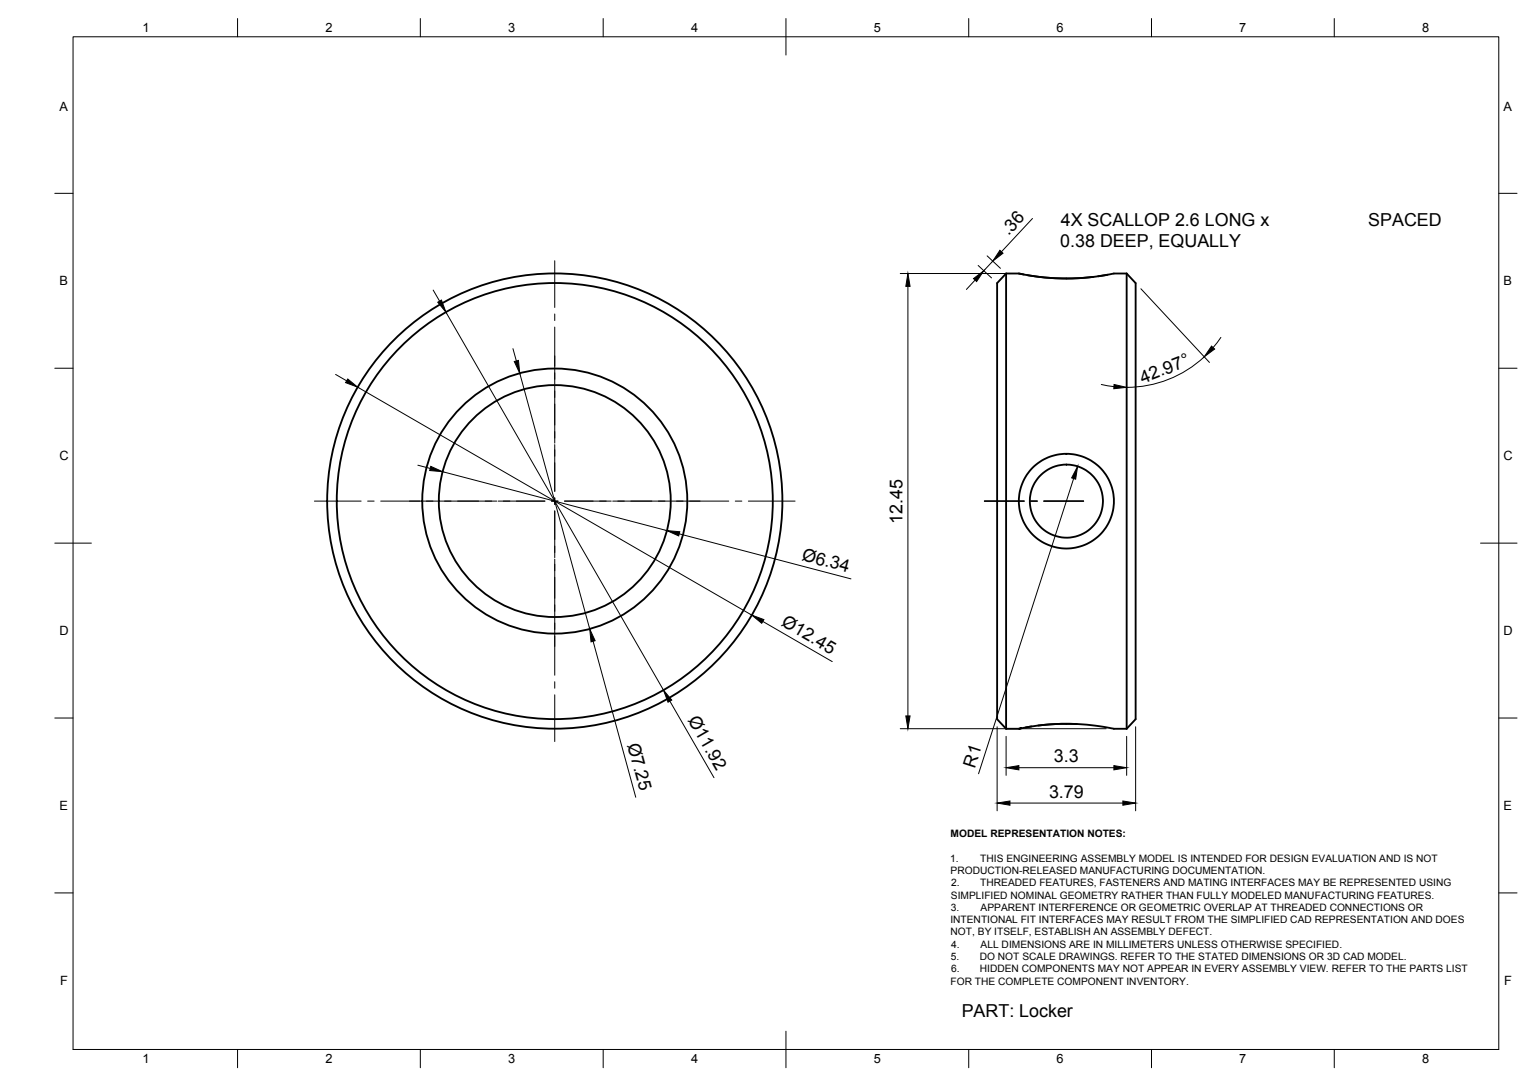
ISO-10303-21;
HEADER;
/* Generated by software containing ST-Developer
 * from STEP Tools, Inc. (www.steptools.com) 
 */

FILE_DESCRIPTION(
/* description */ (''),
/* implementation_level */ '2;1');

FILE_NAME(
/* name */ 'Locker.step',
/* time_stamp */ '2026-10-05T00:51:14-07:00',
/* author */ (''),
/* organization */ (''),
/* preprocessor_version */ 'ST-DEVELOPER v20.2',
/* originating_system */ 'Autodesk Translation Framework v15.15.0.0',
/* authorisation */ '');

FILE_SCHEMA (('AUTOMOTIVE_DESIGN { 1 0 10303 214 3 1 1 }'));
ENDSEC;

DATA;
#10=MECHANICAL_DESIGN_GEOMETRIC_PRESENTATION_REPRESENTATION('',(#392),#4613);
#44=B_SPLINE_SURFACE_WITH_KNOTS('',3,3,((#2717,#2718,#2719,#2720,#2721,
#2722,#2723,#2724,#2725,#2726,#2727,#2728,#2729,#2730,#2731,#2732,#2733,
#2734,#2735,#2736,#2737,#2738,#2739,#2740,#2741,#2742,#2743),(#2744,#2745,
#2746,#2747,#2748,#2749,#2750,#2751,#2752,#2753,#2754,#2755,#2756,#2757,
#2758,#2759,#2760,#2761,#2762,#2763,#2764,#2765,#2766,#2767,#2768,#2769,
#2770),(#2771,#2772,#2773,#2774,#2775,#2776,#2777,#2778,#2779,#2780,#2781,
#2782,#2783,#2784,#2785,#2786,#2787,#2788,#2789,#2790,#2791,#2792,#2793,
#2794,#2795,#2796,#2797),(#2798,#2799,#2800,#2801,#2802,#2803,#2804,#2805,
#2806,#2807,#2808,#2809,#2810,#2811,#2812,#2813,#2814,#2815,#2816,#2817,
#2818,#2819,#2820,#2821,#2822,#2823,#2824)),.UNSPECIFIED.,.F.,.T.,.F.,(4,
4),(4,1,2,1,1,1,2,2,2,2,2,1,1,1,2,2,4),(-9.33776365674593E-5,1.000525980474),
(0.,0.0377394432573701,0.0754788865147403,0.113217461481148,0.150956036447555,
0.188694611413963,0.226433186380371,0.264172629637741,0.301912072895111,
0.339651516152481,0.377390959409851,0.415129534376259,0.452868109342666,
0.490606684309074,0.528345259275481,0.566084702532851,0.603824145790222),
 .UNSPECIFIED.);
#45=B_SPLINE_SURFACE_WITH_KNOTS('',3,3,((#3469,#3470,#3471,#3472,#3473,
#3474,#3475,#3476,#3477,#3478,#3479,#3480,#3481,#3482,#3483,#3484,#3485,
#3486,#3487,#3488,#3489,#3490,#3491,#3492,#3493,#3494,#3495,#3496,#3497),
(#3498,#3499,#3500,#3501,#3502,#3503,#3504,#3505,#3506,#3507,#3508,#3509,
#3510,#3511,#3512,#3513,#3514,#3515,#3516,#3517,#3518,#3519,#3520,#3521,
#3522,#3523,#3524,#3525,#3526),(#3527,#3528,#3529,#3530,#3531,#3532,#3533,
#3534,#3535,#3536,#3537,#3538,#3539,#3540,#3541,#3542,#3543,#3544,#3545,
#3546,#3547,#3548,#3549,#3550,#3551,#3552,#3553,#3554,#3555),(#3556,#3557,
#3558,#3559,#3560,#3561,#3562,#3563,#3564,#3565,#3566,#3567,#3568,#3569,
#3570,#3571,#3572,#3573,#3574,#3575,#3576,#3577,#3578,#3579,#3580,#3581,
#3582,#3583,#3584)),.UNSPECIFIED.,.F.,.T.,.F.,(4,4),(4,1,2,1,2,1,2,2,2,
1,2,1,1,1,1,1,2,2,4),(-0.000295807310057764,1.00205953088178),(0.,0.0377394432573701,
0.0754788865147402,0.113217461481148,0.150956036447555,0.188694611413963,
0.226433186380371,0.264172629637741,0.301912072895111,0.367956098595508,
0.377390959409851,0.415129534376259,0.433998821859462,0.443433465601064,
0.452868109342666,0.490606684309074,0.528345259275481,0.566084702532851,
0.603824145790222),.UNSPECIFIED.);
#46=B_SPLINE_SURFACE_WITH_KNOTS('',3,3,((#3828,#3829,#3830,#3831,#3832,
#3833,#3834,#3835,#3836,#3837,#3838,#3839,#3840,#3841,#3842,#3843,#3844,
#3845,#3846,#3847,#3848,#3849,#3850,#3851,#3852,#3853,#3854),(#3855,#3856,
#3857,#3858,#3859,#3860,#3861,#3862,#3863,#3864,#3865,#3866,#3867,#3868,
#3869,#3870,#3871,#3872,#3873,#3874,#3875,#3876,#3877,#3878,#3879,#3880,
#3881),(#3882,#3883,#3884,#3885,#3886,#3887,#3888,#3889,#3890,#3891,#3892,
#3893,#3894,#3895,#3896,#3897,#3898,#3899,#3900,#3901,#3902,#3903,#3904,
#3905,#3906,#3907,#3908),(#3909,#3910,#3911,#3912,#3913,#3914,#3915,#3916,
#3917,#3918,#3919,#3920,#3921,#3922,#3923,#3924,#3925,#3926,#3927,#3928,
#3929,#3930,#3931,#3932,#3933,#3934,#3935)),.UNSPECIFIED.,.F.,.T.,.F.,(4,
4),(4,1,2,1,1,1,1,2,2,1,1,2,1,1,2,2,2,4),(-0.000127845078603306,1.00073508349094),
(0.,0.0377394432573701,0.0754788865147403,0.113217461481148,0.150956036447555,
0.160390680189157,0.188694611413963,0.226433186380371,0.264172629637741,
0.292477212080768,0.320781794523796,0.377390959409851,0.405694890634657,
0.433998821859462,0.490606684309074,0.528345259275481,0.566084702532852,
0.603824145790222),.UNSPECIFIED.);
#47=B_SPLINE_SURFACE_WITH_KNOTS('',3,3,((#4130,#4131,#4132,#4133,#4134,
#4135,#4136,#4137,#4138,#4139,#4140,#4141,#4142,#4143,#4144,#4145,#4146,
#4147,#4148,#4149,#4150,#4151,#4152,#4153,#4154,#4155,#4156,#4157,#4158,
#4159),(#4160,#4161,#4162,#4163,#4164,#4165,#4166,#4167,#4168,#4169,#4170,
#4171,#4172,#4173,#4174,#4175,#4176,#4177,#4178,#4179,#4180,#4181,#4182,
#4183,#4184,#4185,#4186,#4187,#4188,#4189),(#4190,#4191,#4192,#4193,#4194,
#4195,#4196,#4197,#4198,#4199,#4200,#4201,#4202,#4203,#4204,#4205,#4206,
#4207,#4208,#4209,#4210,#4211,#4212,#4213,#4214,#4215,#4216,#4217,#4218,
#4219),(#4220,#4221,#4222,#4223,#4224,#4225,#4226,#4227,#4228,#4229,#4230,
#4231,#4232,#4233,#4234,#4235,#4236,#4237,#4238,#4239,#4240,#4241,#4242,
#4243,#4244,#4245,#4246,#4247,#4248,#4249)),.UNSPECIFIED.,.F.,.T.,.F.,(4,
4),(4,1,2,1,2,1,2,2,2,2,2,1,1,1,2,2,2,4),(-9.8278797788155E-5,1.00068681548426),
(0.,0.0377394432573701,0.0754788865147402,0.113217461481148,0.150956036447555,
0.188694611413963,0.226433186380371,0.264172629637741,0.301912072895111,
0.339651516152481,0.377390959409851,0.412770873440858,0.433998821859462,
0.462302753084268,0.490606684309074,0.528345259275481,0.566084702532851,
0.603824145790222),.UNSPECIFIED.);
#60=CONICAL_SURFACE('',#1831,6.09377868362497,0.82078898923398);
#61=CONICAL_SURFACE('',#1832,6.09377868362497,0.82078898923398);
#62=CONICAL_SURFACE('',#1836,3.39812786153974,1.04516253667508);
#63=CONICAL_SURFACE('',#1840,3.39812786153974,1.04516253667508);
#84=FACE_BOUND('',#587,.T.);
#85=FACE_BOUND('',#588,.T.);
#86=FACE_BOUND('',#589,.T.);
#87=FACE_BOUND('',#602,.T.);
#88=FACE_BOUND('',#606,.T.);
#114=PLANE('',#1822);
#115=PLANE('',#1823);
#116=PLANE('',#1824);
#117=PLANE('',#1827);
#118=PLANE('',#1828);
#119=PLANE('',#1834);
#139=B_SPLINE_CURVE_WITH_KNOTS('',3,(#2829,#2830,#2831,#2832,#2833,#2834,
#2835,#2836,#2837,#2838,#2839,#2840,#2841,#2842,#2843,#2844,#2845,#2846,
#2847,#2848,#2849,#2850,#2851,#2852,#2853,#2854,#2855,#2856,#2857,#2858,
#2859,#2860,#2861,#2862,#2863,#2864,#2865,#2866,#2867,#2868,#2869,#2870,
#2871,#2872,#2873,#2874,#2875,#2876,#2877,#2878,#2879,#2880,#2881,#2882,
#2883,#2884,#2885,#2886),.UNSPECIFIED.,.F.,.F.,(4,3,3,3,3,3,3,3,3,3,3,3,
3,3,3,3,3,3,3,4),(0.,0.00830256342986541,0.0165421526797814,0.024758238338255,
0.0329694780959283,0.0377394432573701,0.0461457227075515,0.0546067113015583,
0.063111349941413,0.0717202621168138,0.0754788865147403,0.0836526270820083,
0.0917610027075096,0.0998510566328465,0.107954786491979,0.113217461481148,
0.124926744470172,0.136958735315253,0.149276745375588,0.150956036447555),
 .UNSPECIFIED.);
#140=B_SPLINE_CURVE_WITH_KNOTS('',3,(#2887,#2888,#2889,#2890,#2891,#2892,
#2893,#2894,#2895,#2896,#2897,#2898,#2899,#2900,#2901,#2902,#2903,#2904,
#2905,#2906,#2907,#2908),.UNSPECIFIED.,.F.,.F.,(4,1,2,2,2,2,2,1,1,1,2,2,
4),(0.150956036447555,0.188694611413963,0.226433186380371,0.264172629637741,
0.301912072895111,0.339651516152481,0.377390959409851,0.415129534376259,
0.452868109342666,0.490606684309074,0.528345259275481,0.566084702532851,
0.603824145790222),.UNSPECIFIED.);
#141=B_SPLINE_CURVE_WITH_KNOTS('',3,(#2910,#2911,#2912,#2913,#2914,#2915,
#2916,#2917,#2918,#2919,#2920,#2921,#2922,#2923,#2924,#2925,#2926,#2927),
 .UNSPECIFIED.,.F.,.F.,(4,2,2,2,2,2,2,2,4),(0.,0.0225535375719625,0.045742561528813,
0.0614467959049737,0.0822737875323286,0.105553304717535,0.131394096503778,
0.166373424514803,0.179386291539105),.UNSPECIFIED.);
#142=B_SPLINE_CURVE_WITH_KNOTS('',3,(#2929,#2930,#2931,#2932,#2933,#2934,
#2935,#2936,#2937,#2938,#2939,#2940,#2941,#2942,#2943,#2944,#2945,#2946,
#2947,#2948,#2949,#2950,#2951,#2952,#2953,#2954,#2955,#2956,#2957,#2958,
#2959,#2960),.UNSPECIFIED.,.F.,.F.,(4,2,2,2,2,2,2,2,2,2,2,2,2,2,2,4),(0.179386291539105,
0.180187796446041,0.193753938234979,0.227654303126555,0.255593035139534,
0.354710269922964,0.40331380346349,0.454831190769845,0.497871745499511,
0.537911247906565,0.557044545701239,0.596336621939663,0.650672125427441,
0.738536442549073,0.86973485948851,1.00167935296521),.UNSPECIFIED.);
#143=B_SPLINE_CURVE_WITH_KNOTS('',3,(#2961,#2962,#2963,#2964,#2965,#2966,
#2967,#2968,#2969,#2970,#2971,#2972,#2973,#2974),.UNSPECIFIED.,.F.,.F.,
(4,2,2,2,2,2,4),(2.12484122892953E-5,0.0384114166919255,0.0840005064200764,
0.134083217100535,0.322530315130806,0.421641395496061,0.518312663440211),
 .UNSPECIFIED.);
#144=B_SPLINE_CURVE_WITH_KNOTS('',3,(#2983,#2984,#2985,#2986,#2987,#2988,
#2989,#2990,#2991,#2992,#2993,#2994,#2995,#2996,#2997,#2998,#2999,#3000,
#3001,#3002,#3003,#3004,#3005,#3006,#3007,#3008,#3009,#3010,#3011,#3012,
#3013,#3014,#3015,#3016,#3017,#3018,#3019,#3020,#3021,#3022,#3023,#3024,
#3025,#3026,#3027,#3028,#3029,#3030,#3031,#3032,#3033,#3034,#3035,#3036,
#3037,#3038,#3039,#3040,#3041,#3042,#3043,#3044,#3045,#3046,#3047,#3048,
#3049,#3050,#3051,#3052,#3053,#3054,#3055,#3056,#3057,#3058,#3059,#3060,
#3061,#3062,#3063,#3064,#3065,#3066,#3067,#3068,#3069,#3070,#3071,#3072,
#3073,#3074,#3075,#3076,#3077,#3078,#3079,#3080,#3081,#3082,#3083,#3084,
#3085,#3086,#3087,#3088,#3089,#3090,#3091,#3092,#3093,#3094,#3095,#3096,
#3097,#3098,#3099,#3100,#3101,#3102,#3103,#3104,#3105,#3106,#3107,#3108,
#3109,#3110,#3111,#3112,#3113,#3114,#3115,#3116,#3117,#3118,#3119,#3120,
#3121,#3122,#3123,#3124,#3125,#3126,#3127,#3128,#3129,#3130,#3131,#3132,
#3133,#3134,#3135,#3136,#3137,#3138,#3139,#3140,#3141,#3142,#3143,#3144,
#3145,#3146,#3147,#3148),.UNSPECIFIED.,.T.,.F.,(4,3,3,3,3,3,3,3,3,3,3,3,
3,3,3,3,3,3,3,3,3,3,3,3,3,3,3,3,3,3,3,3,3,3,3,3,3,3,3,3,3,3,3,3,3,3,3,3,
3,3,3,3,3,3,3,4),(-0.603824145790222,-0.590391584697042,-0.577063699872746,
-0.566084702532851,-0.547214980904166,-0.533196018247437,-0.528345259275481,
-0.514141540772843,-0.5016291634541,-0.490606684309074,-0.479313082523423,
-0.468129273627917,-0.456937255878014,-0.452868109342666,-0.44488880016883,
-0.443433465601064,-0.43506567000572,-0.433998821859462,-0.422340513015576,
-0.415129534376259,-0.402742107601763,-0.388956278039157,-0.377390959409851,
-0.368495774245557,-0.367956098595508,-0.35039657661204,-0.334829325286879,
-0.320458700988321,-0.307238340240676,-0.301912072895111,-0.288351696410483,
-0.275229547002117,-0.264172629637741,-0.245302908009056,-0.231165617978299,
-0.226433186380371,-0.211738883366401,-0.19886806654317,-0.188694611413963,
-0.177840892685696,-0.167083403070668,-0.156287372800931,-0.150956036447555,
-0.140167573510221,-0.129416044354867,-0.118538583805277,-0.113217461481148,
-0.100521490014891,-0.0863362768838805,-0.0754788865147402,-0.0614072540763898,
-0.0441325663214528,-0.0377394432573701,-0.0243206710161803,-0.0108972336665805,
0.),.UNSPECIFIED.);
#145=B_SPLINE_CURVE_WITH_KNOTS('',3,(#3150,#3151,#3152,#3153,#3154,#3155,
#3156,#3157,#3158,#3159,#3160,#3161,#3162,#3163,#3164,#3165,#3166,#3167,
#3168,#3169,#3170,#3171,#3172,#3173,#3174,#3175,#3176,#3177,#3178,#3179,
#3180,#3181,#3182,#3183,#3184,#3185,#3186,#3187,#3188,#3189,#3190,#3191,
#3192,#3193,#3194,#3195,#3196,#3197,#3198,#3199,#3200,#3201,#3202,#3203,
#3204,#3205,#3206,#3207,#3208,#3209,#3210,#3211,#3212,#3213,#3214,#3215,
#3216,#3217,#3218,#3219,#3220,#3221,#3222,#3223,#3224,#3225,#3226,#3227,
#3228,#3229,#3230,#3231,#3232,#3233,#3234,#3235,#3236,#3237,#3238,#3239,
#3240,#3241,#3242,#3243,#3244,#3245,#3246,#3247,#3248,#3249,#3250,#3251,
#3252,#3253,#3254,#3255,#3256,#3257,#3258,#3259,#3260,#3261,#3262,#3263,
#3264,#3265,#3266,#3267,#3268,#3269,#3270,#3271,#3272,#3273,#3274,#3275,
#3276,#3277,#3278,#3279,#3280,#3281,#3282,#3283,#3284,#3285,#3286,#3287,
#3288,#3289,#3290,#3291,#3292,#3293,#3294,#3295,#3296,#3297,#3298,#3299,
#3300,#3301,#3302,#3303,#3304,#3305,#3306),.UNSPECIFIED.,.T.,.F.,(4,3,3,
3,3,3,3,3,3,3,3,3,3,3,3,3,3,3,3,3,3,3,3,3,3,3,3,3,3,3,3,3,3,3,3,3,3,3,3,
3,3,3,3,3,3,3,3,3,3,3,3,3,4),(-0.603824145790222,-0.59040484149205,-0.577046286087289,
-0.566084702532851,-0.547214980904166,-0.533215939038458,-0.528345259275481,
-0.513405700683712,-0.500371614295665,-0.490606684309074,-0.479523112948318,
-0.468575947550825,-0.462302753084268,-0.448150787471865,-0.433998821859462,
-0.424198693428956,-0.414259352480831,-0.412770873440858,-0.398547629668401,
-0.382168241492649,-0.377390959409851,-0.363265067662413,-0.345806810116418,
-0.339651516152481,-0.326317147459025,-0.312908174453228,-0.301912072895111,
-0.288487301763661,-0.2751501468201,-0.264172629637741,-0.245302908009056,
-0.231228232357298,-0.226433186380371,-0.2117347177624,-0.198863361209748,
-0.188694611413963,-0.177846084312265,-0.167093676385978,-0.15630237051341,
-0.150956036447555,-0.140168989421454,-0.129419180679109,-0.118543795278154,
-0.113217461481148,-0.10052665633752,-0.0863472586539609,-0.0754788865147402,
-0.0614129693111486,-0.0441577717811917,-0.0377394432573701,-0.0243211983180093,
-0.0108969351998749,0.),.UNSPECIFIED.);
#146=B_SPLINE_CURVE_WITH_KNOTS('',3,(#3308,#3309,#3310,#3311,#3312,#3313,
#3314,#3315,#3316,#3317,#3318,#3319,#3320,#3321,#3322,#3323,#3324,#3325,
#3326,#3327,#3328,#3329,#3330,#3331,#3332,#3333,#3334,#3335,#3336,#3337,
#3338,#3339,#3340,#3341,#3342,#3343,#3344,#3345,#3346,#3347,#3348,#3349,
#3350,#3351,#3352,#3353,#3354,#3355,#3356,#3357,#3358,#3359,#3360,#3361,
#3362,#3363,#3364,#3365,#3366,#3367,#3368,#3369,#3370,#3371,#3372,#3373,
#3374,#3375,#3376,#3377,#3378,#3379,#3380,#3381,#3382,#3383,#3384,#3385,
#3386,#3387,#3388,#3389,#3390,#3391,#3392,#3393,#3394,#3395,#3396,#3397,
#3398,#3399,#3400,#3401,#3402,#3403,#3404,#3405,#3406,#3407,#3408,#3409,
#3410,#3411,#3412,#3413,#3414,#3415,#3416,#3417,#3418,#3419,#3420,#3421,
#3422,#3423,#3424,#3425,#3426,#3427,#3428,#3429,#3430,#3431,#3432,#3433,
#3434,#3435,#3436,#3437,#3438,#3439,#3440,#3441,#3442,#3443,#3444,#3445,
#3446,#3447,#3448,#3449,#3450,#3451,#3452,#3453,#3454,#3455,#3456,#3457,
#3458,#3459,#3460,#3461,#3462,#3463,#3464),.UNSPECIFIED.,.T.,.F.,(4,3,3,
3,3,3,3,3,3,3,3,3,3,3,3,3,3,3,3,3,3,3,3,3,3,3,3,3,3,3,3,3,3,3,3,3,3,3,3,
3,3,3,3,3,3,3,3,3,3,3,3,3,4),(-0.603824145790222,-0.590411465612469,-0.577041801624018,
-0.566084702532852,-0.547214980904167,-0.533151553554515,-0.528345259275481,
-0.511854870778258,-0.497832584846173,-0.490606684309074,-0.473210539692822,
-0.455925683856001,-0.438701796249427,-0.433998821859462,-0.423201659387045,
-0.412132127313061,-0.405694890634657,-0.390813405226797,-0.377390959409851,
-0.359294156561789,-0.340037975542793,-0.32497088632671,-0.320781794523796,
-0.307843399048729,-0.294273409598876,-0.292477212080768,-0.279144117317815,
-0.266288363724764,-0.264172629637741,-0.245302908009056,-0.231166470585065,
-0.226433186380371,-0.210823746419028,-0.197307415534654,-0.188694611413963,
-0.178396491003475,-0.168205689857489,-0.160390680189157,-0.15167832823336,
-0.150956036447555,-0.139587056809165,-0.128218450390218,-0.116689538696443,
-0.113217461481148,-0.100992605061081,-0.0874389990760216,-0.0754788865147403,
-0.0614233370420267,-0.0442069385936118,-0.0377394432573701,-0.0243181691647032,
-0.010894129954878,0.),.UNSPECIFIED.);
#147=B_SPLINE_CURVE_WITH_KNOTS('',3,(#3588,#3589,#3590,#3591,#3592,#3593,
#3594,#3595,#3596,#3597,#3598,#3599,#3600,#3601,#3602,#3603,#3604,#3605,
#3606,#3607,#3608,#3609,#3610,#3611,#3612,#3613,#3614,#3615,#3616,#3617,
#3618,#3619,#3620,#3621,#3622,#3623,#3624,#3625,#3626,#3627,#3628,#3629,
#3630,#3631,#3632,#3633,#3634,#3635,#3636,#3637,#3638,#3639,#3640,#3641,
#3642,#3643,#3644,#3645),.UNSPECIFIED.,.F.,.F.,(4,3,3,3,3,3,3,3,3,3,3,3,
3,3,3,3,3,3,3,4),(0.,0.00829573762667763,0.0165281897599753,0.0247370376512881,
0.0329409858379027,0.0377394432573701,0.0462233213317535,0.0547599525540828,
0.0633384602639499,0.0720158188648333,0.0754788865147402,0.0849135302563422,
0.0940108607641121,0.103092592101262,0.112175512163797,0.113217461481148,
0.122710740047244,0.132228579300877,0.141826740872809,0.150956036447555),
 .UNSPECIFIED.);
#148=B_SPLINE_CURVE_WITH_KNOTS('',3,(#3646,#3647,#3648,#3649,#3650,#3651,
#3652,#3653,#3654,#3655,#3656,#3657,#3658,#3659,#3660,#3661,#3662,#3663,
#3664,#3665,#3666,#3667,#3668,#3669,#3670,#3671,#3672,#3673,#3674,#3675,
#3676,#3677,#3678,#3679,#3680,#3681,#3682,#3683,#3684,#3685,#3686,#3687,
#3688,#3689,#3690,#3691,#3692,#3693,#3694,#3695,#3696,#3697,#3698,#3699,
#3700,#3701,#3702,#3703,#3704,#3705,#3706,#3707,#3708,#3709,#3710,#3711,
#3712,#3713,#3714,#3715,#3716,#3717,#3718,#3719,#3720,#3721,#3722,#3723,
#3724,#3725,#3726,#3727,#3728,#3729,#3730,#3731,#3732,#3733,#3734,#3735,
#3736,#3737,#3738,#3739,#3740,#3741,#3742,#3743,#3744,#3745,#3746,#3747,
#3748,#3749,#3750,#3751,#3752,#3753,#3754,#3755,#3756,#3757,#3758,#3759,
#3760,#3761,#3762,#3763,#3764,#3765,#3766,#3767,#3768,#3769,#3770,#3771,
#3772,#3773,#3774,#3775,#3776,#3777,#3778,#3779,#3780,#3781,#3782,#3783,
#3784,#3785,#3786,#3787,#3788,#3789,#3790,#3791,#3792,#3793,#3794,#3795,
#3796,#3797,#3798,#3799,#3800,#3801,#3802,#3803,#3804,#3805,#3806,#3807,
#3808,#3809,#3810,#3811,#3812,#3813,#3814,#3815,#3816,#3817,#3818,#3819,
#3820,#3821,#3822,#3823),.UNSPECIFIED.,.F.,.F.,(4,3,3,3,3,3,3,3,3,3,3,3,
3,3,3,3,3,3,3,3,3,3,3,3,3,3,3,3,3,3,3,3,3,3,3,3,3,3,3,3,3,3,3,3,3,3,3,3,
3,3,3,3,3,3,3,3,3,3,3,4),(0.150956036447555,0.160549363754181,0.170087496495515,
0.17957549259755,0.188694611413963,0.198129255155565,0.20721232152291,0.216307090036003,
0.225442296384496,0.226433186380371,0.235263130335913,0.243982144413462,
0.252652316208085,0.261280881376461,0.264172629637741,0.272628973289914,
0.281096319050457,0.289577868539869,0.298109252272672,0.301912072895111,
0.310541878044286,0.3191353238789,0.327707744142598,0.336272944326547,0.344860159102294,
0.35346693169753,0.362137437500319,0.367956098595508,0.375378363711079,
0.377390959409851,0.386825603151453,0.395781405680958,0.404721766264308,
0.413665159126656,0.415129534376259,0.426960243388473,0.433998821859462,
0.440518945174589,0.443433465601064,0.449108910733518,0.452868109342666,
0.463354416125425,0.473794794225623,0.484190742563337,0.490606684309074,
0.499415552802534,0.508224959525105,0.517045112657598,0.525909821728332,
0.528345259275481,0.537116996273335,0.545776074243873,0.554386030522553,
0.562954515301158,0.566084702532851,0.574305585613258,0.582536335557294,
0.590782316872269,0.59908512911533,0.603824145790222),.UNSPECIFIED.);
#149=B_SPLINE_CURVE_WITH_KNOTS('',3,(#3939,#3940,#3941,#3942,#3943,#3944,
#3945,#3946,#3947,#3948,#3949,#3950,#3951,#3952,#3953,#3954,#3955,#3956),
 .UNSPECIFIED.,.F.,.F.,(4,2,2,2,2,2,2,2,4),(-0.157966795349973,-0.134769746245384,
-0.111152103192473,-0.0957393456100155,-0.0764377111352473,-0.0499851580328299,
-0.0372293294602945,-0.0183607331665397,-1.54852585271355E-5),
 .UNSPECIFIED.);
#150=B_SPLINE_CURVE_WITH_KNOTS('',3,(#3957,#3958,#3959,#3960,#3961,#3962,
#3963,#3964,#3965,#3966,#3967,#3968,#3969,#3970,#3971,#3972,#3973,#3974,
#3975,#3976,#3977,#3978,#3979,#3980,#3981,#3982,#3983,#3984,#3985,#3986,
#3987,#3988,#3989,#3990,#3991,#3992,#3993,#3994,#3995,#3996,#3997,#3998,
#3999,#4000,#4001,#4002,#4003,#4004,#4005,#4006,#4007,#4008,#4009,#4010,
#4011,#4012,#4013,#4014,#4015,#4016,#4017,#4018,#4019,#4020,#4021,#4022,
#4023,#4024,#4025,#4026,#4027,#4028,#4029,#4030,#4031,#4032,#4033,#4034,
#4035,#4036,#4037,#4038,#4039,#4040,#4041,#4042,#4043,#4044,#4045,#4046,
#4047,#4048,#4049,#4050,#4051,#4052,#4053,#4054,#4055,#4056,#4057,#4058,
#4059,#4060,#4061,#4062,#4063,#4064,#4065,#4066,#4067,#4068,#4069,#4070,
#4071,#4072,#4073,#4074,#4075,#4076,#4077,#4078,#4079,#4080,#4081,#4082,
#4083,#4084,#4085,#4086,#4087,#4088,#4089,#4090,#4091,#4092,#4093,#4094,
#4095,#4096,#4097,#4098,#4099,#4100,#4101,#4102,#4103,#4104,#4105,#4106,
#4107,#4108,#4109,#4110,#4111,#4112,#4113,#4114,#4115,#4116,#4117,#4118,
#4119,#4120,#4121,#4122),.UNSPECIFIED.,.F.,.F.,(4,3,3,3,3,3,3,3,3,3,3,3,
3,3,3,3,3,3,3,3,3,3,3,3,3,3,3,3,3,3,3,3,3,3,3,3,3,3,3,3,3,3,3,3,3,3,3,3,
3,3,3,3,3,3,3,4),(0.150956046102631,0.157057308185334,0.160390680189157,
0.169102327349017,0.177761740636142,0.186381822627463,0.188694611413963,
0.198129255155565,0.207504363975699,0.216968775178035,0.226433186380371,
0.235339806064433,0.244136369675249,0.252883841436447,0.26158882295505,
0.264172629637741,0.273921145643219,0.283689652217834,0.292477212080768,
0.301909496950062,0.311349416446087,0.320781794523796,0.328948709583596,
0.33710056797636,0.345254117291374,0.353452734644994,0.361688284787263,
0.37003334621096,0.377390959409851,0.385901375718853,0.394375368564309,
0.402830843321504,0.405694890634657,0.415170724108714,0.424683263298954,
0.433998821859462,0.443965968418747,0.454061131183995,0.46415325099199,
0.474130092027922,0.483814161418412,0.490606684309074,0.500095510584781,
0.509588520092461,0.519121097655791,0.528345259275481,0.537152260065718,
0.545849424317997,0.554498405743932,0.563106711158609,0.566084702532852,
0.574301473245816,0.582528508095237,0.590771006435055,0.599070784708944,
0.603824145790222),.UNSPECIFIED.);
#151=B_SPLINE_CURVE_WITH_KNOTS('',3,(#4253,#4254,#4255,#4256,#4257,#4258,
#4259,#4260,#4261,#4262,#4263,#4264,#4265,#4266,#4267,#4268,#4269,#4270,
#4271,#4272),.UNSPECIFIED.,.F.,.F.,(4,2,2,2,2,2,2,2,2,4),(-0.63257270273012,
-0.613187885769762,-0.594110099534741,-0.574392662092664,-0.55480528669817,
-0.535546049297075,-0.516021545010237,-0.496492553321205,-0.477063998339651,
-0.474227533561733),.UNSPECIFIED.);
#152=B_SPLINE_CURVE_WITH_KNOTS('',3,(#4273,#4274,#4275,#4276,#4277,#4278,
#4279,#4280,#4281,#4282,#4283,#4284,#4285,#4286,#4287,#4288,#4289,#4290,
#4291,#4292,#4293,#4294,#4295,#4296,#4297,#4298,#4299,#4300,#4301,#4302,
#4303,#4304,#4305,#4306,#4307,#4308,#4309,#4310,#4311,#4312,#4313,#4314,
#4315,#4316,#4317,#4318,#4319,#4320,#4321,#4322,#4323,#4324),
 .UNSPECIFIED.,.F.,.F.,(4,2,2,2,2,2,2,2,2,2,2,2,2,2,2,2,2,2,2,2,2,2,2,2,
2,4),(-0.474227533561733,-0.458329372527362,-0.439173439486182,-0.419731155843369,
-0.400140639763559,-0.381254494509653,-0.362129574615996,-0.342849277390761,
-0.315940533098414,-0.289017768986139,-0.269733478910581,-0.250586364422205,
-0.231653812692583,-0.21172855838034,-0.201929598171686,-0.182564500685825,
-0.163995370742465,-0.144570150007686,-0.125002244985411,-0.105396599383871,
-0.0956567919090896,-0.0764809925540918,-0.0569765610843296,-0.0373737466489288,
-0.0184652873791742,0.),.UNSPECIFIED.);
#205=LINE('',#2827,#288);
#206=LINE('',#2978,#289);
#207=LINE('',#2980,#290);
#208=LINE('',#3468,#291);
#209=LINE('',#3586,#292);
#210=LINE('',#3827,#293);
#211=LINE('',#3937,#294);
#212=LINE('',#4126,#295);
#213=LINE('',#4251,#296);
#214=LINE('',#4328,#297);
#215=LINE('',#4336,#298);
#216=LINE('',#4339,#299);
#217=LINE('',#4347,#300);
#218=LINE('',#4351,#301);
#219=LINE('',#4353,#302);
#288=VECTOR('',#2186,10.);
#289=VECTOR('',#2191,6.22506754791384);
#290=VECTOR('',#2192,6.22506754791384);
#291=VECTOR('',#2199,1.);
#292=VECTOR('',#2200,9.99999999999999);
#293=VECTOR('',#2205,1.);
#294=VECTOR('',#2206,10.);
#295=VECTOR('',#2211,1.);
#296=VECTOR('',#2218,10.);
#297=VECTOR('',#2223,1.);
#298=VECTOR('',#2234,6.09377868362497);
#299=VECTOR('',#2237,6.09377868362497);
#300=VECTOR('',#2248,3.39812786153974);
#301=VECTOR('',#2253,3.17127539348974);
#302=VECTOR('',#2256,3.39812786153974);
#354=CYLINDRICAL_SURFACE('',#1813,6.22506754791384);
#355=CYLINDRICAL_SURFACE('',#1816,1.);
#356=CYLINDRICAL_SURFACE('',#1818,1.);
#357=CYLINDRICAL_SURFACE('',#1820,1.);
#358=CYLINDRICAL_SURFACE('',#1825,1.);
#359=CYLINDRICAL_SURFACE('',#1838,3.17127539348974);
#376=SHAPE_REPRESENTATION_RELATIONSHIP('SRR','None',#4650,#384);
#384=ADVANCED_BREP_SHAPE_REPRESENTATION('',(#400),#4610);
#392=STYLED_ITEM('',(#4695),#400);
#400=MANIFOLD_SOLID_BREP('Body1',#1599);
#462=FACE_OUTER_BOUND('',#585,.T.);
#463=FACE_OUTER_BOUND('',#586,.T.);
#464=FACE_OUTER_BOUND('',#590,.T.);
#465=FACE_OUTER_BOUND('',#591,.T.);
#466=FACE_OUTER_BOUND('',#592,.T.);
#467=FACE_OUTER_BOUND('',#593,.T.);
#468=FACE_OUTER_BOUND('',#594,.T.);
#469=FACE_OUTER_BOUND('',#595,.T.);
#470=FACE_OUTER_BOUND('',#596,.T.);
#471=FACE_OUTER_BOUND('',#597,.T.);
#472=FACE_OUTER_BOUND('',#598,.T.);
#473=FACE_OUTER_BOUND('',#599,.T.);
#474=FACE_OUTER_BOUND('',#600,.T.);
#475=FACE_OUTER_BOUND('',#601,.T.);
#476=FACE_OUTER_BOUND('',#603,.T.);
#477=FACE_OUTER_BOUND('',#604,.T.);
#478=FACE_OUTER_BOUND('',#605,.T.);
#479=FACE_OUTER_BOUND('',#607,.T.);
#480=FACE_OUTER_BOUND('',#608,.T.);
#481=FACE_OUTER_BOUND('',#609,.T.);
#585=EDGE_LOOP('',(#1277,#1278,#1279,#1280,#1281,#1282,#1283));
#586=EDGE_LOOP('',(#1284,#1285,#1286,#1287,#1288,#1289,#1290,#1291,#1292));
#587=EDGE_LOOP('',(#1293));
#588=EDGE_LOOP('',(#1294));
#589=EDGE_LOOP('',(#1295));
#590=EDGE_LOOP('',(#1296,#1297,#1298,#1299,#1300));
#591=EDGE_LOOP('',(#1301,#1302,#1303,#1304,#1305));
#592=EDGE_LOOP('',(#1306,#1307,#1308,#1309,#1310));
#593=EDGE_LOOP('',(#1311,#1312,#1313,#1314,#1315));
#594=EDGE_LOOP('',(#1316,#1317,#1318,#1319,#1320));
#595=EDGE_LOOP('',(#1321));
#596=EDGE_LOOP('',(#1322));
#597=EDGE_LOOP('',(#1323));
#598=EDGE_LOOP('',(#1324,#1325,#1326,#1327,#1328));
#599=EDGE_LOOP('',(#1329,#1330,#1331,#1332,#1333));
#600=EDGE_LOOP('',(#1334));
#601=EDGE_LOOP('',(#1335));
#602=EDGE_LOOP('',(#1336));
#603=EDGE_LOOP('',(#1337,#1338,#1339,#1340));
#604=EDGE_LOOP('',(#1341,#1342,#1343,#1344));
#605=EDGE_LOOP('',(#1345));
#606=EDGE_LOOP('',(#1346));
#607=EDGE_LOOP('',(#1347,#1348,#1349,#1350));
#608=EDGE_LOOP('',(#1351,#1352,#1353,#1354));
#609=EDGE_LOOP('',(#1355,#1356,#1357,#1358));
#695=CIRCLE('',#1814,6.22506754791384);
#696=CIRCLE('',#1815,6.22506754791384);
#697=CIRCLE('',#1817,1.);
#698=CIRCLE('',#1819,1.);
#699=CIRCLE('',#1821,1.);
#700=CIRCLE('',#1826,1.);
#701=CIRCLE('',#1829,5.96248981933611);
#702=CIRCLE('',#1830,3.62498032958974);
#703=CIRCLE('',#1833,5.96248981933611);
#704=CIRCLE('',#1835,3.62498032958974);
#705=CIRCLE('',#1837,3.17127539348974);
#706=CIRCLE('',#1839,3.17127539348974);
#796=VERTEX_POINT('',#2825);
#797=VERTEX_POINT('',#2826);
#798=VERTEX_POINT('',#2828);
#799=VERTEX_POINT('',#2909);
#800=VERTEX_POINT('',#2928);
#801=VERTEX_POINT('',#2976);
#802=VERTEX_POINT('',#2979);
#803=VERTEX_POINT('',#2982);
#804=VERTEX_POINT('',#3149);
#805=VERTEX_POINT('',#3307);
#806=VERTEX_POINT('',#3466);
#807=VERTEX_POINT('',#3585);
#808=VERTEX_POINT('',#3587);
#809=VERTEX_POINT('',#3825);
#810=VERTEX_POINT('',#3936);
#811=VERTEX_POINT('',#3938);
#812=VERTEX_POINT('',#4124);
#813=VERTEX_POINT('',#4250);
#814=VERTEX_POINT('',#4252);
#815=VERTEX_POINT('',#4326);
#816=VERTEX_POINT('',#4331);
#817=VERTEX_POINT('',#4333);
#818=VERTEX_POINT('',#4338);
#819=VERTEX_POINT('',#4342);
#820=VERTEX_POINT('',#4345);
#821=VERTEX_POINT('',#4349);
#966=EDGE_CURVE('',#796,#797,#205,.T.);
#967=EDGE_CURVE('',#797,#798,#139,.T.);
#968=EDGE_CURVE('',#798,#797,#140,.T.);
#969=EDGE_CURVE('',#796,#799,#141,.T.);
#970=EDGE_CURVE('',#799,#800,#142,.T.);
#971=EDGE_CURVE('',#800,#796,#143,.T.);
#972=EDGE_CURVE('',#801,#801,#695,.T.);
#973=EDGE_CURVE('',#801,#799,#206,.T.);
#974=EDGE_CURVE('',#800,#802,#207,.T.);
#975=EDGE_CURVE('',#802,#802,#696,.T.);
#976=EDGE_CURVE('',#803,#803,#144,.T.);
#977=EDGE_CURVE('',#804,#804,#145,.T.);
#978=EDGE_CURVE('',#805,#805,#146,.T.);
#979=EDGE_CURVE('',#806,#806,#697,.T.);
#980=EDGE_CURVE('',#806,#798,#208,.T.);
#981=EDGE_CURVE('',#803,#807,#209,.T.);
#982=EDGE_CURVE('',#807,#808,#147,.T.);
#983=EDGE_CURVE('',#808,#807,#148,.T.);
#984=EDGE_CURVE('',#809,#809,#698,.T.);
#985=EDGE_CURVE('',#809,#808,#210,.T.);
#986=EDGE_CURVE('',#805,#810,#211,.T.);
#987=EDGE_CURVE('',#810,#811,#149,.T.);
#988=EDGE_CURVE('',#811,#810,#150,.T.);
#989=EDGE_CURVE('',#812,#812,#699,.T.);
#990=EDGE_CURVE('',#812,#811,#212,.T.);
#991=EDGE_CURVE('',#804,#813,#213,.T.);
#992=EDGE_CURVE('',#813,#814,#151,.T.);
#993=EDGE_CURVE('',#814,#813,#152,.T.);
#994=EDGE_CURVE('',#815,#815,#700,.T.);
#995=EDGE_CURVE('',#815,#814,#214,.T.);
#996=EDGE_CURVE('',#816,#816,#701,.T.);
#997=EDGE_CURVE('',#817,#817,#702,.T.);
#998=EDGE_CURVE('',#802,#816,#215,.T.);
#999=EDGE_CURVE('',#801,#818,#216,.T.);
#1000=EDGE_CURVE('',#818,#818,#703,.T.);
#1001=EDGE_CURVE('',#819,#819,#704,.T.);
#1002=EDGE_CURVE('',#820,#820,#705,.T.);
#1003=EDGE_CURVE('',#820,#819,#217,.T.);
#1004=EDGE_CURVE('',#821,#821,#706,.T.);
#1005=EDGE_CURVE('',#821,#820,#218,.T.);
#1006=EDGE_CURVE('',#821,#817,#219,.T.);
#1277=ORIENTED_EDGE('',*,*,#966,.T.);
#1278=ORIENTED_EDGE('',*,*,#967,.T.);
#1279=ORIENTED_EDGE('',*,*,#968,.T.);
#1280=ORIENTED_EDGE('',*,*,#966,.F.);
#1281=ORIENTED_EDGE('',*,*,#969,.T.);
#1282=ORIENTED_EDGE('',*,*,#970,.T.);
#1283=ORIENTED_EDGE('',*,*,#971,.T.);
#1284=ORIENTED_EDGE('',*,*,#972,.F.);
#1285=ORIENTED_EDGE('',*,*,#973,.T.);
#1286=ORIENTED_EDGE('',*,*,#969,.F.);
#1287=ORIENTED_EDGE('',*,*,#971,.F.);
#1288=ORIENTED_EDGE('',*,*,#974,.T.);
#1289=ORIENTED_EDGE('',*,*,#975,.T.);
#1290=ORIENTED_EDGE('',*,*,#974,.F.);
#1291=ORIENTED_EDGE('',*,*,#970,.F.);
#1292=ORIENTED_EDGE('',*,*,#973,.F.);
#1293=ORIENTED_EDGE('',*,*,#976,.F.);
#1294=ORIENTED_EDGE('',*,*,#977,.F.);
#1295=ORIENTED_EDGE('',*,*,#978,.F.);
#1296=ORIENTED_EDGE('',*,*,#979,.F.);
#1297=ORIENTED_EDGE('',*,*,#980,.T.);
#1298=ORIENTED_EDGE('',*,*,#967,.F.);
#1299=ORIENTED_EDGE('',*,*,#968,.F.);
#1300=ORIENTED_EDGE('',*,*,#980,.F.);
#1301=ORIENTED_EDGE('',*,*,#981,.T.);
#1302=ORIENTED_EDGE('',*,*,#982,.T.);
#1303=ORIENTED_EDGE('',*,*,#983,.T.);
#1304=ORIENTED_EDGE('',*,*,#981,.F.);
#1305=ORIENTED_EDGE('',*,*,#976,.T.);
#1306=ORIENTED_EDGE('',*,*,#984,.F.);
#1307=ORIENTED_EDGE('',*,*,#985,.T.);
#1308=ORIENTED_EDGE('',*,*,#982,.F.);
#1309=ORIENTED_EDGE('',*,*,#983,.F.);
#1310=ORIENTED_EDGE('',*,*,#985,.F.);
#1311=ORIENTED_EDGE('',*,*,#986,.T.);
#1312=ORIENTED_EDGE('',*,*,#987,.T.);
#1313=ORIENTED_EDGE('',*,*,#988,.T.);
#1314=ORIENTED_EDGE('',*,*,#986,.F.);
#1315=ORIENTED_EDGE('',*,*,#978,.T.);
#1316=ORIENTED_EDGE('',*,*,#989,.F.);
#1317=ORIENTED_EDGE('',*,*,#990,.T.);
#1318=ORIENTED_EDGE('',*,*,#987,.F.);
#1319=ORIENTED_EDGE('',*,*,#988,.F.);
#1320=ORIENTED_EDGE('',*,*,#990,.F.);
#1321=ORIENTED_EDGE('',*,*,#979,.T.);
#1322=ORIENTED_EDGE('',*,*,#984,.T.);
#1323=ORIENTED_EDGE('',*,*,#989,.T.);
#1324=ORIENTED_EDGE('',*,*,#991,.T.);
#1325=ORIENTED_EDGE('',*,*,#992,.T.);
#1326=ORIENTED_EDGE('',*,*,#993,.T.);
#1327=ORIENTED_EDGE('',*,*,#991,.F.);
#1328=ORIENTED_EDGE('',*,*,#977,.T.);
#1329=ORIENTED_EDGE('',*,*,#994,.F.);
#1330=ORIENTED_EDGE('',*,*,#995,.T.);
#1331=ORIENTED_EDGE('',*,*,#992,.F.);
#1332=ORIENTED_EDGE('',*,*,#993,.F.);
#1333=ORIENTED_EDGE('',*,*,#995,.F.);
#1334=ORIENTED_EDGE('',*,*,#994,.T.);
#1335=ORIENTED_EDGE('',*,*,#996,.F.);
#1336=ORIENTED_EDGE('',*,*,#997,.T.);
#1337=ORIENTED_EDGE('',*,*,#975,.F.);
#1338=ORIENTED_EDGE('',*,*,#998,.T.);
#1339=ORIENTED_EDGE('',*,*,#996,.T.);
#1340=ORIENTED_EDGE('',*,*,#998,.F.);
#1341=ORIENTED_EDGE('',*,*,#972,.T.);
#1342=ORIENTED_EDGE('',*,*,#999,.T.);
#1343=ORIENTED_EDGE('',*,*,#1000,.F.);
#1344=ORIENTED_EDGE('',*,*,#999,.F.);
#1345=ORIENTED_EDGE('',*,*,#1000,.T.);
#1346=ORIENTED_EDGE('',*,*,#1001,.F.);
#1347=ORIENTED_EDGE('',*,*,#1002,.F.);
#1348=ORIENTED_EDGE('',*,*,#1003,.T.);
#1349=ORIENTED_EDGE('',*,*,#1001,.T.);
#1350=ORIENTED_EDGE('',*,*,#1003,.F.);
#1351=ORIENTED_EDGE('',*,*,#1004,.F.);
#1352=ORIENTED_EDGE('',*,*,#1005,.T.);
#1353=ORIENTED_EDGE('',*,*,#1002,.T.);
#1354=ORIENTED_EDGE('',*,*,#1005,.F.);
#1355=ORIENTED_EDGE('',*,*,#1004,.T.);
#1356=ORIENTED_EDGE('',*,*,#1006,.T.);
#1357=ORIENTED_EDGE('',*,*,#997,.F.);
#1358=ORIENTED_EDGE('',*,*,#1006,.F.);
#1547=ADVANCED_FACE('',(#462),#44,.T.);
#1548=ADVANCED_FACE('',(#463,#84,#85,#86),#354,.T.);
#1549=ADVANCED_FACE('',(#464),#355,.F.);
#1550=ADVANCED_FACE('',(#465),#45,.T.);
#1551=ADVANCED_FACE('',(#466),#356,.F.);
#1552=ADVANCED_FACE('',(#467),#46,.T.);
#1553=ADVANCED_FACE('',(#468),#357,.F.);
#1554=ADVANCED_FACE('',(#469),#114,.F.);
#1555=ADVANCED_FACE('',(#470),#115,.F.);
#1556=ADVANCED_FACE('',(#471),#116,.F.);
#1557=ADVANCED_FACE('',(#472),#47,.T.);
#1558=ADVANCED_FACE('',(#473),#358,.F.);
#1559=ADVANCED_FACE('',(#474),#117,.F.);
#1560=ADVANCED_FACE('',(#475,#87),#118,.T.);
#1561=ADVANCED_FACE('',(#476),#60,.T.);
#1562=ADVANCED_FACE('',(#477),#61,.T.);
#1563=ADVANCED_FACE('',(#478,#88),#119,.T.);
#1564=ADVANCED_FACE('',(#479),#62,.F.);
#1565=ADVANCED_FACE('',(#480),#359,.F.);
#1566=ADVANCED_FACE('',(#481),#63,.F.);
#1599=CLOSED_SHELL('',(#1547,#1548,#1549,#1550,#1551,#1552,#1553,#1554,
#1555,#1556,#1557,#1558,#1559,#1560,#1561,#1562,#1563,#1564,#1565,#1566));
#1812=AXIS2_PLACEMENT_3D('',#2716,#2184,#2185);
#1813=AXIS2_PLACEMENT_3D('',#2975,#2187,#2188);
#1814=AXIS2_PLACEMENT_3D('',#2977,#2189,#2190);
#1815=AXIS2_PLACEMENT_3D('',#2981,#2193,#2194);
#1816=AXIS2_PLACEMENT_3D('',#3465,#2195,#2196);
#1817=AXIS2_PLACEMENT_3D('',#3467,#2197,#2198);
#1818=AXIS2_PLACEMENT_3D('',#3824,#2201,#2202);
#1819=AXIS2_PLACEMENT_3D('',#3826,#2203,#2204);
#1820=AXIS2_PLACEMENT_3D('',#4123,#2207,#2208);
#1821=AXIS2_PLACEMENT_3D('',#4125,#2209,#2210);
#1822=AXIS2_PLACEMENT_3D('',#4127,#2212,#2213);
#1823=AXIS2_PLACEMENT_3D('',#4128,#2214,#2215);
#1824=AXIS2_PLACEMENT_3D('',#4129,#2216,#2217);
#1825=AXIS2_PLACEMENT_3D('',#4325,#2219,#2220);
#1826=AXIS2_PLACEMENT_3D('',#4327,#2221,#2222);
#1827=AXIS2_PLACEMENT_3D('',#4329,#2224,#2225);
#1828=AXIS2_PLACEMENT_3D('',#4330,#2226,#2227);
#1829=AXIS2_PLACEMENT_3D('',#4332,#2228,#2229);
#1830=AXIS2_PLACEMENT_3D('',#4334,#2230,#2231);
#1831=AXIS2_PLACEMENT_3D('',#4335,#2232,#2233);
#1832=AXIS2_PLACEMENT_3D('',#4337,#2235,#2236);
#1833=AXIS2_PLACEMENT_3D('',#4340,#2238,#2239);
#1834=AXIS2_PLACEMENT_3D('',#4341,#2240,#2241);
#1835=AXIS2_PLACEMENT_3D('',#4343,#2242,#2243);
#1836=AXIS2_PLACEMENT_3D('',#4344,#2244,#2245);
#1837=AXIS2_PLACEMENT_3D('',#4346,#2246,#2247);
#1838=AXIS2_PLACEMENT_3D('',#4348,#2249,#2250);
#1839=AXIS2_PLACEMENT_3D('',#4350,#2251,#2252);
#1840=AXIS2_PLACEMENT_3D('',#4352,#2254,#2255);
#2184=DIRECTION('axis',(0.,0.,1.));
#2185=DIRECTION('refdir',(1.,0.,0.));
#2186=DIRECTION('',(0.,0.769537968693233,-0.638601060709652));
#2187=DIRECTION('center_axis',(1.,0.,0.));
#2188=DIRECTION('ref_axis',(0.,0.,-1.));
#2189=DIRECTION('center_axis',(1.,0.,0.));
#2190=DIRECTION('ref_axis',(0.,0.,-1.));
#2191=DIRECTION('',(-1.,0.,0.));
#2192=DIRECTION('',(-1.,0.,0.));
#2193=DIRECTION('center_axis',(1.,0.,0.));
#2194=DIRECTION('ref_axis',(0.,0.,-1.));
#2195=DIRECTION('center_axis',(0.,1.83697019872103E-16,1.));
#2196=DIRECTION('ref_axis',(1.,0.,0.));
#2197=DIRECTION('center_axis',(0.,1.83697019872103E-16,1.));
#2198=DIRECTION('ref_axis',(1.,0.,0.));
#2199=DIRECTION('',(0.,1.83697019872103E-16,1.));
#2200=DIRECTION('',(0.,-0.63860106070965,-0.769537968693234));
#2201=DIRECTION('center_axis',(0.,1.,-1.22464679914735E-16));
#2202=DIRECTION('ref_axis',(1.,0.,0.));
#2203=DIRECTION('center_axis',(0.,1.,-1.22464679914735E-16));
#2204=DIRECTION('ref_axis',(1.,0.,0.));
#2205=DIRECTION('',(0.,1.,-1.22464679914735E-16));
#2206=DIRECTION('',(0.,-0.769537968693233,0.638601060709652));
#2207=DIRECTION('center_axis',(0.,-6.12323399573677E-17,-1.));
#2208=DIRECTION('ref_axis',(1.,0.,0.));
#2209=DIRECTION('center_axis',(0.,-6.12323399573677E-17,-1.));
#2210=DIRECTION('ref_axis',(1.,0.,0.));
#2211=DIRECTION('',(0.,-6.12323399573677E-17,-1.));
#2212=DIRECTION('center_axis',(0.,-1.83697019872103E-16,-1.));
#2213=DIRECTION('ref_axis',(1.,0.,0.));
#2214=DIRECTION('center_axis',(0.,-1.,1.22464679914735E-16));
#2215=DIRECTION('ref_axis',(1.,0.,0.));
#2216=DIRECTION('center_axis',(0.,6.12323399573677E-17,1.));
#2217=DIRECTION('ref_axis',(1.,0.,0.));
#2218=DIRECTION('',(0.,0.638601060709651,0.769537968693234));
#2219=DIRECTION('center_axis',(0.,-1.,0.));
#2220=DIRECTION('ref_axis',(1.,0.,0.));
#2221=DIRECTION('center_axis',(0.,-1.,0.));
#2222=DIRECTION('ref_axis',(1.,0.,0.));
#2223=DIRECTION('',(0.,-1.,0.));
#2224=DIRECTION('center_axis',(0.,1.,0.));
#2225=DIRECTION('ref_axis',(1.,0.,0.));
#2226=DIRECTION('center_axis',(-1.,0.,0.));
#2227=DIRECTION('ref_axis',(0.,0.,1.));
#2228=DIRECTION('center_axis',(1.,0.,0.));
#2229=DIRECTION('ref_axis',(0.,0.,-1.));
#2230=DIRECTION('center_axis',(1.,0.,0.));
#2231=DIRECTION('ref_axis',(0.,0.,-1.));
#2232=DIRECTION('center_axis',(1.,0.,0.));
#2233=DIRECTION('ref_axis',(0.,0.,-1.));
#2234=DIRECTION('',(-0.681644128816632,8.9605430606225E-17,-0.731683867288199));
#2235=DIRECTION('center_axis',(-1.,0.,0.));
#2236=DIRECTION('ref_axis',(0.,0.,-1.));
#2237=DIRECTION('',(0.681644128816632,-8.9605430606225E-17,-0.731683867288199));
#2238=DIRECTION('center_axis',(1.,0.,0.));
#2239=DIRECTION('ref_axis',(0.,0.,-1.));
#2240=DIRECTION('center_axis',(1.,0.,0.));
#2241=DIRECTION('ref_axis',(0.,0.,-1.));
#2242=DIRECTION('center_axis',(1.,0.,0.));
#2243=DIRECTION('ref_axis',(0.,0.,-1.));
#2244=DIRECTION('center_axis',(1.,0.,0.));
#2245=DIRECTION('ref_axis',(0.,0.,-1.));
#2246=DIRECTION('center_axis',(1.,0.,0.));
#2247=DIRECTION('ref_axis',(0.,0.,-1.));
#2248=DIRECTION('',(0.501761337735621,-1.05932695650405E-16,0.865006103997978));
#2249=DIRECTION('center_axis',(1.,0.,0.));
#2250=DIRECTION('ref_axis',(0.,0.,-1.));
#2251=DIRECTION('center_axis',(1.,0.,0.));
#2252=DIRECTION('ref_axis',(0.,0.,-1.));
#2253=DIRECTION('',(1.,0.,0.));
#2254=DIRECTION('center_axis',(-1.,0.,0.));
#2255=DIRECTION('ref_axis',(0.,0.,-1.));
#2256=DIRECTION('',(-0.501761337735621,1.05932695650405E-16,0.865006103997978));
#2716=CARTESIAN_POINT('',(0.,0.,0.));
#2717=CARTESIAN_POINT('Ctrl Pts',(-12.4302293937643,-1.29488419085615,6.08893179912409));
#2718=CARTESIAN_POINT('Ctrl Pts',(-12.5942554551731,-1.29488414718856,6.08893179050175));
#2719=CARTESIAN_POINT('Ctrl Pts',(-12.9434041993798,-1.2294328459869,6.10376298255976));
#2720=CARTESIAN_POINT('Ctrl Pts',(-13.2352719744654,-1.0316590890245,6.14035711678102));
#2721=CARTESIAN_POINT('Ctrl Pts',(-13.4652582677038,-0.804188184632238,
6.1743411575965));
#2722=CARTESIAN_POINT('Ctrl Pts',(-13.6645706157926,-0.50626213886193,6.21083535170997));
#2723=CARTESIAN_POINT('Ctrl Pts',(-13.7634101258885,-4.55193504007075E-5,
6.23259369899848));
#2724=CARTESIAN_POINT('Ctrl Pts',(-13.6645494097846,0.506350803091124,6.21079370032761));
#2725=CARTESIAN_POINT('Ctrl Pts',(-13.4651211785068,0.804025993881401,6.17427297012694));
#2726=CARTESIAN_POINT('Ctrl Pts',(-13.2354048303999,1.03253237976219,6.14014393621034));
#2727=CARTESIAN_POINT('Ctrl Pts',(-13.0895391630103,1.13181896559648,6.12197280773622));
#2728=CARTESIAN_POINT('Ctrl Pts',(-12.7690246025484,1.26358725386243,6.09603285881286));
#2729=CARTESIAN_POINT('Ctrl Pts',(-12.5943534667659,1.29612320858372,6.08887111511598));
#2730=CARTESIAN_POINT('Ctrl Pts',(-12.2661214257273,1.29612709871105,6.08886919819022));
#2731=CARTESIAN_POINT('Ctrl Pts',(-12.0914504696733,1.26359486961962,6.09602904830329));
#2732=CARTESIAN_POINT('Ctrl Pts',(-11.7709375208824,1.13183595785232,6.12196443982891));
#2733=CARTESIAN_POINT('Ctrl Pts',(-11.6250715919502,1.03254971804437,6.14013512447093));
#2734=CARTESIAN_POINT('Ctrl Pts',(-11.395360898952,0.804063499952342,6.17425479916453));
#2735=CARTESIAN_POINT('Ctrl Pts',(-11.1959336454396,0.506396277936275,6.2107637521937));
#2736=CARTESIAN_POINT('Ctrl Pts',(-11.0970937797084,6.1156379640301E-5,
6.23254880516501));
#2737=CARTESIAN_POINT('Ctrl Pts',(-11.1959237146699,-0.506186673149979,
6.21076962890895));
#2738=CARTESIAN_POINT('Ctrl Pts',(-11.3952900549715,-0.803952284531892,
6.17425879944784));
#2739=CARTESIAN_POINT('Ctrl Pts',(-11.6251494839037,-1.03184033349927,6.14017845211199));
#2740=CARTESIAN_POINT('Ctrl Pts',(-11.7709627360902,-1.13109996217884,6.12198310555546));
#2741=CARTESIAN_POINT('Ctrl Pts',(-12.0914571818659,-1.26265113550208,6.09609663062554));
#2742=CARTESIAN_POINT('Ctrl Pts',(-12.2662033433641,-1.29488420847439,6.08893179144279));
#2743=CARTESIAN_POINT('Ctrl Pts',(-12.4302293937643,-1.29488419085615,6.08893179912409));
#2744=CARTESIAN_POINT('Ctrl Pts',(-12.4302293937643,-1.19653776428921,6.00731901992712));
#2745=CARTESIAN_POINT('Ctrl Pts',(-12.5835320638101,-1.19669374251964,6.00734981845634));
#2746=CARTESIAN_POINT('Ctrl Pts',(-12.9098993488334,-1.13385554423326,6.02032135745683));
#2747=CARTESIAN_POINT('Ctrl Pts',(-13.1794444923897,-0.948175876780826,
6.05212160800709));
#2748=CARTESIAN_POINT('Ctrl Pts',(-13.3904188730421,-0.736106912634719,
6.08151671837308));
#2749=CARTESIAN_POINT('Ctrl Pts',(-13.571358399148,-0.461107396153454,6.11288518823509));
#2750=CARTESIAN_POINT('Ctrl Pts',(-13.6598647804087,-4.77349200694727E-5,
6.13145209579345));
#2751=CARTESIAN_POINT('Ctrl Pts',(-13.5713351984267,0.461201603549934,6.11284433707963));
#2752=CARTESIAN_POINT('Ctrl Pts',(-13.3902865479058,0.73593723140633,6.0814466719145));
#2753=CARTESIAN_POINT('Ctrl Pts',(-13.1795657386676,0.949053789500503,6.05191117775911));
#2754=CARTESIAN_POINT('Ctrl Pts',(-13.0448959816465,1.04218619158655,6.03613258011903));
#2755=CARTESIAN_POINT('Ctrl Pts',(-12.7468860466288,1.16681531246955,6.01352866653896));
#2756=CARTESIAN_POINT('Ctrl Pts',(-12.5836668315555,1.19776542529252,6.00726540810815));
#2757=CARTESIAN_POINT('Ctrl Pts',(-12.2768080336065,1.19776973044414,6.00726351057582));
#2758=CARTESIAN_POINT('Ctrl Pts',(-12.1135891439065,1.16682230335479,6.01352482644386));
#2759=CARTESIAN_POINT('Ctrl Pts',(-11.8155804810902,1.04220414880451,6.03612425707734));
#2760=CARTESIAN_POINT('Ctrl Pts',(-11.6809112042485,0.949069004361932,6.05190226572165));
#2761=CARTESIAN_POINT('Ctrl Pts',(-11.4701945190351,0.735978790867167,6.08142869039248));
#2762=CARTESIAN_POINT('Ctrl Pts',(-11.2891496988235,0.461239711890714,6.11281404103072));
#2763=CARTESIAN_POINT('Ctrl Pts',(-11.2006363964354,6.98177936070269E-5,
6.13140771052673));
#2764=CARTESIAN_POINT('Ctrl Pts',(-11.2891410326498,-0.461052166154195,
6.11281851072142));
#2765=CARTESIAN_POINT('Ctrl Pts',(-11.4701207397339,-0.735837035061057,
6.08143595189992));
#2766=CARTESIAN_POINT('Ctrl Pts',(-11.6809938866623,-0.948407049105129,
6.05194059445036));
#2767=CARTESIAN_POINT('Ctrl Pts',(-11.8156020963373,-1.04142835561581,6.03614993606957));
#2768=CARTESIAN_POINT('Ctrl Pts',(-12.1135988587321,-1.16591750294593,6.01358226833267));
#2769=CARTESIAN_POINT('Ctrl Pts',(-12.2768874021684,-1.1964748328885,6.00734645713312));
#2770=CARTESIAN_POINT('Ctrl Pts',(-12.4302293937643,-1.19653776428921,6.00731901992712));
#2771=CARTESIAN_POINT('Ctrl Pts',(-12.4302293937643,-1.09819133772228,5.92570624073015));
#2772=CARTESIAN_POINT('Ctrl Pts',(-12.5728763428205,-1.09803515711868,5.92567540224153));
#2773=CARTESIAN_POINT('Ctrl Pts',(-12.876321077954,-1.0387969727173,5.93681987239533));
#2774=CARTESIAN_POINT('Ctrl Pts',(-13.1236914762163,-0.863950043440302,
5.96385707568949));
#2775=CARTESIAN_POINT('Ctrl Pts',(-13.3155790887801,-0.668255697608592,
5.98863521528464));
#2776=CARTESIAN_POINT('Ctrl Pts',(-13.4781865651095,-0.415776757496831,
6.0149151254311));
#2777=CARTESIAN_POINT('Ctrl Pts',(-13.5561689964186,4.21654537423543E-5,
6.03022023183205));
#2778=CARTESIAN_POINT('Ctrl Pts',(-13.478150753931,0.415977680530914,6.01488398902043));
#2779=CARTESIAN_POINT('Ctrl Pts',(-13.315393862027,0.668313266257187,5.98858257490239));
#2780=CARTESIAN_POINT('Ctrl Pts',(-13.1237891612582,0.864807186170974,5.96371046903562));
#2781=CARTESIAN_POINT('Ctrl Pts',(-13.000238685325,0.952440693384399,5.95029853437126));
#2782=CARTESIAN_POINT('Ctrl Pts',(-12.7247805462859,1.06962276776914,5.93103239143954));
#2783=CARTESIAN_POINT('Ctrl Pts',(-12.5729657038671,1.09913712296315,5.92566846199632));
#2784=CARTESIAN_POINT('Ctrl Pts',(-12.2875198521031,1.09913697678003,5.92566694755825));
#2785=CARTESIAN_POINT('Ctrl Pts',(-12.1357051736444,1.06962385288842,5.93102945126453));
#2786=CARTESIAN_POINT('Ctrl Pts',(-11.8602500197414,0.952440909619879,5.95029196307193));
#2787=CARTESIAN_POINT('Ctrl Pts',(-11.7366984580338,0.864810198814481,5.96370370664712));
#2788=CARTESIAN_POINT('Ctrl Pts',(-11.5451044624593,0.668312166922651,5.98856820249765));
#2789=CARTESIAN_POINT('Ctrl Pts',(-11.3823489586879,0.415979415085571,6.01486124976089));
#2790=CARTESIAN_POINT('Ctrl Pts',(-11.3043647489821,4.76005030248672E-5,
6.0301844356551));
#2791=CARTESIAN_POINT('Ctrl Pts',(-11.3823356020908,-0.415784531254904,
6.0148658425333));
#2792=CARTESIAN_POINT('Ctrl Pts',(-11.5450254725926,-0.66823389832439,5.98856817993586));
#2793=CARTESIAN_POINT('Ctrl Pts',(-11.7367782945029,-0.864224843995978,
5.96372965668036));
#2794=CARTESIAN_POINT('Ctrl Pts',(-11.8602868211275,-0.951940725192759,
5.9502902505237));
#2795=CARTESIAN_POINT('Ctrl Pts',(-12.1357015099293,-1.06885043095419,5.9310779680282));
#2796=CARTESIAN_POINT('Ctrl Pts',(-12.2876218172759,-1.09825435077303,5.92567876792588));
#2797=CARTESIAN_POINT('Ctrl Pts',(-12.4302293937643,-1.09819133772228,5.92570624073015));
#2798=CARTESIAN_POINT('Ctrl Pts',(-12.4302293937643,-0.999844911155348,
5.84409346153317));
#2799=CARTESIAN_POINT('Ctrl Pts',(-12.5621528929196,-0.999845157446748,
5.8440935101644));
#2800=CARTESIAN_POINT('Ctrl Pts',(-12.8428162909195,-0.943219222239121,
5.85337829907391));
#2801=CARTESIAN_POINT('Ctrl Pts',(-13.0678639297245,-0.780467473596644,
5.87562159202221));
#2802=CARTESIAN_POINT('Ctrl Pts',(-13.2407396944553,-0.600174226601641,
5.89581082542398));
#2803=CARTESIAN_POINT('Ctrl Pts',(-13.3849743135323,-0.370622166946112,
5.91696497917002));
#2804=CARTESIAN_POINT('Ctrl Pts',(-13.4526237810749,3.98701997180173E-5,
5.92907870670656));
#2805=CARTESIAN_POINT('Ctrl Pts',(-13.3849365168234,0.370828545628829,5.9169346352748));
#2806=CARTESIAN_POINT('Ctrl Pts',(-13.2405592816462,0.60022410171192,5.89575630938757));
#2807=CARTESIAN_POINT('Ctrl Pts',(-13.0679500154482,0.781329260274485,5.87547768285996));
#2808=CARTESIAN_POINT('Ctrl Pts',(-12.9555955161712,0.862808016885863,5.86445830140649));
#2809=CARTESIAN_POINT('Ctrl Pts',(-12.7026419617718,0.972851190216686,5.84852819231695));
#2810=CARTESIAN_POINT('Ctrl Pts',(-12.5622790811935,1.00077957368287,5.84406274740993));
#2811=CARTESIAN_POINT('Ctrl Pts',(-12.2982064381739,1.00077984673363,5.84406125205068));
#2812=CARTESIAN_POINT('Ctrl Pts',(-12.157843867466,0.972851655032226,5.84852522175233));
#2813=CARTESIAN_POINT('Ctrl Pts',(-11.9048929569576,0.862809214264935,5.86445177349625));
#2814=CARTESIAN_POINT('Ctrl Pts',(-11.7925381156245,0.781330158215836,5.87547081822711));
#2815=CARTESIAN_POINT('Ctrl Pts',(-11.6199380165194,0.600227096175383,5.89574212346506));
#2816=CARTESIAN_POINT('Ctrl Pts',(-11.4755650265989,0.370822938771694,5.91691154126233));
#2817=CARTESIAN_POINT('Ctrl Pts',(-11.4079072050394,5.62886284334987E-5,
5.92904341210635));
#2818=CARTESIAN_POINT('Ctrl Pts',(-11.4755529397492,-0.370650139420631,
5.91691472568658));
#2819=CARTESIAN_POINT('Ctrl Pts',(-11.6198560933002,-0.600118205853443,
5.89574537124953));
#2820=CARTESIAN_POINT('Ctrl Pts',(-11.7926227491599,-0.780792207451304,
5.87549177573183));
#2821=CARTESIAN_POINT('Ctrl Pts',(-11.9049261421322,-0.862268959482245,
5.86445710397538));
#2822=CARTESIAN_POINT('Ctrl Pts',(-12.1578432205544,-0.972117086837851,
5.84856359703126));
#2823=CARTESIAN_POINT('Ctrl Pts',(-12.2983058325198,-0.99984481178595,5.84409350485683));
#2824=CARTESIAN_POINT('Ctrl Pts',(-12.4302293937643,-0.999844911155348,
5.84409346153317));
#2825=CARTESIAN_POINT('',(-12.4302293937643,-1.29485665783831,6.08890895085005));
#2826=CARTESIAN_POINT('',(-12.4302293937643,-1.,5.84422216200635));
#2827=CARTESIAN_POINT('',(-12.4302293937643,-1.29485665783831,6.08890895085005));
#2828=CARTESIAN_POINT('',(-13.4302255152826,6.09774944770533E-5,5.92519355911023));
#2829=CARTESIAN_POINT('Ctrl Pts',(-12.4302293937643,-0.999999999999999,
5.84422216200635));
#2830=CARTESIAN_POINT('Ctrl Pts',(-12.4592558850193,-0.999999999999999,
5.84422216200635));
#2831=CARTESIAN_POINT('Ctrl Pts',(-12.488694554397,-0.998732061148834,5.84444691869061));
#2832=CARTESIAN_POINT('Ctrl Pts',(-12.5183095428325,-0.996113390804545,
5.84488149270083));
#2833=CARTESIAN_POINT('Ctrl Pts',(-12.5476999043046,-0.993514582833954,
5.84531277050715));
#2834=CARTESIAN_POINT('Ctrl Pts',(-12.5772632652184,-0.989585307459082,
5.84595069482016));
#2835=CARTESIAN_POINT('Ctrl Pts',(-12.6067599503988,-0.984295160292032,
5.84678066365066));
#2836=CARTESIAN_POINT('Ctrl Pts',(-12.6361724957008,-0.979020103374498,
5.84760826497863));
#2837=CARTESIAN_POINT('Ctrl Pts',(-12.6655180670433,-0.972391909338808,
5.84862681676514));
#2838=CARTESIAN_POINT('Ctrl Pts',(-12.6945598901648,-0.964432158667805,
5.84982184162226));
#2839=CARTESIAN_POINT('Ctrl Pts',(-12.7235845842301,-0.956477102709557,
5.85101616164594));
#2840=CARTESIAN_POINT('Ctrl Pts',(-12.7523052168835,-0.947192192568073,
5.85238674663169));
#2841=CARTESIAN_POINT('Ctrl Pts',(-12.7804964410769,-0.936649878859193,
5.85391914479304));
#2842=CARTESIAN_POINT('Ctrl Pts',(-12.7968729154253,-0.930525776945672,
5.85480932533323));
#2843=CARTESIAN_POINT('Ctrl Pts',(-12.8130709993127,-0.923978305979963,
5.85575411017152));
#2844=CARTESIAN_POINT('Ctrl Pts',(-12.8290495544449,-0.917029159533509,
5.85675066634454));
#2845=CARTESIAN_POINT('Ctrl Pts',(-12.8572091311095,-0.90478243130972,5.85850693277305));
#2846=CARTESIAN_POINT('Ctrl Pts',(-12.8847319564144,-0.89126554770641,5.86042399200011));
#2847=CARTESIAN_POINT('Ctrl Pts',(-12.9114199263146,-0.876616034181418,
5.86245467738282));
#2848=CARTESIAN_POINT('Ctrl Pts',(-12.9382815849427,-0.861871179745247,
5.86449857872621));
#2849=CARTESIAN_POINT('Ctrl Pts',(-12.9642969455781,-0.845979342985271,
5.86665759002513));
#2850=CARTESIAN_POINT('Ctrl Pts',(-12.9892973901898,-0.829121809731686,
5.86888361773069));
#2851=CARTESIAN_POINT('Ctrl Pts',(-13.0144268115212,-0.812177308851183,
5.87112112946207));
#2852=CARTESIAN_POINT('Ctrl Pts',(-13.0385304149824,-0.794257687420666,
5.87342635085594));
#2853=CARTESIAN_POINT('Ctrl Pts',(-13.0614777313691,-0.775580773531183,
5.87575044017624));
#2854=CARTESIAN_POINT('Ctrl Pts',(-13.0847063998404,-0.7566748660387,5.87810302465319));
#2855=CARTESIAN_POINT('Ctrl Pts',(-13.1067499553324,-0.73699361188813,5.88047494256405));
#2856=CARTESIAN_POINT('Ctrl Pts',(-13.12752017916,-0.716788365281066,5.88281553354217));
#2857=CARTESIAN_POINT('Ctrl Pts',(-13.1365883945672,-0.707966817178806,
5.88383742831548));
#2858=CARTESIAN_POINT('Ctrl Pts',(-13.1454145186503,-0.699045653989259,
5.88485335164735));
#2859=CARTESIAN_POINT('Ctrl Pts',(-13.1539941405822,-0.690046803676091,
5.88585908744382));
#2860=CARTESIAN_POINT('Ctrl Pts',(-13.1726519250301,-0.670477338872932,
5.88804622364294));
#2861=CARTESIAN_POINT('Ctrl Pts',(-13.1907859755752,-0.64986192549443,5.89025601762883));
#2862=CARTESIAN_POINT('Ctrl Pts',(-13.2081852637323,-0.628318919325442,
5.89245033006015));
#2863=CARTESIAN_POINT('Ctrl Pts',(-13.2254454107646,-0.606948191360311,
5.89462709469886));
#2864=CARTESIAN_POINT('Ctrl Pts',(-13.2419819765234,-0.584665033083303,
5.89678862440316));
#2865=CARTESIAN_POINT('Ctrl Pts',(-13.2576215487824,-0.561624627143889,
5.89889768752854));
#2866=CARTESIAN_POINT('Ctrl Pts',(-13.2732257818358,-0.538636283347225,
5.90100198501107));
#2867=CARTESIAN_POINT('Ctrl Pts',(-13.2879366304041,-0.514894595696598,
5.90305405275394));
#2868=CARTESIAN_POINT('Ctrl Pts',(-13.301621703492,-0.490586834869639,5.90501691092882));
#2869=CARTESIAN_POINT('Ctrl Pts',(-13.3153299106845,-0.466237982681504,
5.90698308724208));
#2870=CARTESIAN_POINT('Ctrl Pts',(-13.3280085421283,-0.441321716069898,
5.90885975212154));
#2871=CARTESIAN_POINT('Ctrl Pts',(-13.3395704076334,-0.416051583935773,
5.91060973788262));
#2872=CARTESIAN_POINT('Ctrl Pts',(-13.3470788440547,-0.399640808321703,
5.91174620299885));
#2873=CARTESIAN_POINT('Ctrl Pts',(-13.3541172575866,-0.38308129324033,5.91282924266107));
#2874=CARTESIAN_POINT('Ctrl Pts',(-13.3606728897663,-0.366435397781884,
5.9138486772792));
#2875=CARTESIAN_POINT('Ctrl Pts',(-13.3752589610175,-0.32939881449871,5.91611688659423));
#2876=CARTESIAN_POINT('Ctrl Pts',(-13.3874617255085,-0.291938214172012,
5.91807022026964));
#2877=CARTESIAN_POINT('Ctrl Pts',(-13.3973781083062,-0.254211258523014,
5.91968556259891));
#2878=CARTESIAN_POINT('Ctrl Pts',(-13.4075677866282,-0.215444547921944,
5.9213454237651));
#2879=CARTESIAN_POINT('Ctrl Pts',(-13.4153439945548,-0.17639549147079,5.9226484067786));
#2880=CARTESIAN_POINT('Ctrl Pts',(-13.4207734325054,-0.137195143188463,
5.92356943156943));
#2881=CARTESIAN_POINT('Ctrl Pts',(-13.4263319366763,-0.0970629414001139,
5.92451235055809));
#2882=CARTESIAN_POINT('Ctrl Pts',(-13.4294312404248,-0.0567708233405655,
5.92505493599733));
#2883=CARTESIAN_POINT('Ctrl Pts',(-13.4300942971141,-0.0164370024408991,
5.92517027638565));
#2884=CARTESIAN_POINT('Ctrl Pts',(-13.4301846903816,-0.0109383687327478,
5.92518600052318));
#2885=CARTESIAN_POINT('Ctrl Pts',(-13.430229727278,-0.00543894523112027,
5.92519378415999));
#2886=CARTESIAN_POINT('Ctrl Pts',(-13.4302293919052,6.09777308642567E-5,
5.92519355911023));
#2887=CARTESIAN_POINT('Ctrl Pts',(-13.4302255152826,6.09774944770533E-5,
5.92519355911023));
#2888=CARTESIAN_POINT('Ctrl Pts',(-13.4302192163544,0.123659830589739,5.92518850158483));
#2889=CARTESIAN_POINT('Ctrl Pts',(-13.3850835123617,0.370899744283506,5.91708909795873));
#2890=CARTESIAN_POINT('Ctrl Pts',(-13.2406772931872,0.600331475536471,5.89590269316437));
#2891=CARTESIAN_POINT('Ctrl Pts',(-13.0680380717591,0.781460902655162,5.87561682282398));
#2892=CARTESIAN_POINT('Ctrl Pts',(-12.9556659168855,0.862949364547602,5.86459366841997));
#2893=CARTESIAN_POINT('Ctrl Pts',(-12.702676873511,0.973003795928843,5.84865829852133));
#2894=CARTESIAN_POINT('Ctrl Pts',(-12.5622959336324,1.00093468029201,5.8441914367352));
#2895=CARTESIAN_POINT('Ctrl Pts',(-12.2981895857838,1.00093495268569,5.84418994134556));
#2896=CARTESIAN_POINT('Ctrl Pts',(-12.1578089555458,0.97300426172696,5.84865532800387));
#2897=CARTESIAN_POINT('Ctrl Pts',(-11.9048225565987,0.862950560394959,5.86458714043989));
#2898=CARTESIAN_POINT('Ctrl Pts',(-11.7924500584981,0.781461803939683,5.8756099583505));
#2899=CARTESIAN_POINT('Ctrl Pts',(-11.6198200065818,0.6003344635829,5.89588850694494));
#2900=CARTESIAN_POINT('Ctrl Pts',(-11.4754180281628,0.370894149027576,5.91706600449914));
#2901=CARTESIAN_POINT('Ctrl Pts',(-11.4077439220855,5.62749531760182E-5,
5.929202908));
#2902=CARTESIAN_POINT('Ctrl Pts',(-11.4754059393156,-0.370721314874449,
5.91706919114304));
#2903=CARTESIAN_POINT('Ctrl Pts',(-11.6197380879902,-0.600225621472355,
5.89589174958094));
#2904=CARTESIAN_POINT('Ctrl Pts',(-11.7925346844751,-0.780923778396437,
5.87563092373439));
#2905=CARTESIAN_POINT('Ctrl Pts',(-11.9048557474604,-0.862410368540219,
5.86459245984095));
#2906=CARTESIAN_POINT('Ctrl Pts',(-12.1578083038904,-0.972269632184938,
5.84869371927455));
#2907=CARTESIAN_POINT('Ctrl Pts',(-12.298288984163,-1.,5.84422216200635));
#2908=CARTESIAN_POINT('Ctrl Pts',(-12.4302293937643,-1.,5.84422216200635));
#2909=CARTESIAN_POINT('',(-11.1302593513097,-3.3449167263952E-15,6.22506754791384));
#2910=CARTESIAN_POINT('Ctrl Pts',(-12.4302293937643,-1.29485665783831,6.08890895085005));
#2911=CARTESIAN_POINT('Ctrl Pts',(-12.3550509351911,-1.29485665783831,6.08890895085005));
#2912=CARTESIAN_POINT('Ctrl Pts',(-12.2791894522468,-1.28803385899595,6.09037004805683));
#2913=CARTESIAN_POINT('Ctrl Pts',(-12.1289044531663,-1.26195566431335,6.09582777868059));
#2914=CARTESIAN_POINT('Ctrl Pts',(-12.0533392104996,-1.24213987866781,6.09994033109874));
#2915=CARTESIAN_POINT('Ctrl Pts',(-11.9315538541034,-1.19807725994036,6.10871557265866));
#2916=CARTESIAN_POINT('Ctrl Pts',(-11.8841287877011,-1.17740270840153,6.1127532723677));
#2917=CARTESIAN_POINT('Ctrl Pts',(-11.7773853504172,-1.12312910404621,6.12299260884751));
#2918=CARTESIAN_POINT('Ctrl Pts',(-11.7187497040409,-1.08726612645883,6.12951525526529));
#2919=CARTESIAN_POINT('Ctrl Pts',(-11.6017107249225,-1.00275397201799,6.14393994768209));
#2920=CARTESIAN_POINT('Ctrl Pts',(-11.5425195814749,-0.951920261192589,
6.15210896307454));
#2921=CARTESIAN_POINT('Ctrl Pts',(-11.430697412608,-0.835085988005597,6.16911299212126));
#2922=CARTESIAN_POINT('Ctrl Pts',(-11.3777994433336,-0.766398454187795,
6.17813694724593));
#2923=CARTESIAN_POINT('Ctrl Pts',(-11.270636406155,-0.596492970430275,6.19720348504624));
#2924=CARTESIAN_POINT('Ctrl Pts',(-11.1895796685093,-0.441508390314537,
6.21286406982716));
#2925=CARTESIAN_POINT('Ctrl Pts',(-11.1373062258032,-0.156727656024724,
6.22357399872114));
#2926=CARTESIAN_POINT('Ctrl Pts',(-11.1302626056501,-0.0783821040661418,
6.22506754791384));
#2927=CARTESIAN_POINT('Ctrl Pts',(-11.1302593513097,-3.34492582124604E-15,
6.22506754791384));
#2928=CARTESIAN_POINT('',(-13.730193598416,-1.52223171728111E-5,6.22506754789523));
#2929=CARTESIAN_POINT('Ctrl Pts',(-11.1302593513097,-3.34492582124604E-15,
6.22506754791384));
#2930=CARTESIAN_POINT('Ctrl Pts',(-11.1302591508642,0.00482780934498283,
6.22506754791384));
#2931=CARTESIAN_POINT('Ctrl Pts',(-11.1302855894096,0.00965575735666793,
6.22506193146085));
#2932=CARTESIAN_POINT('Ctrl Pts',(-11.1312380214286,0.0961986804474738,
6.22486057533084));
#2933=CARTESIAN_POINT('Ctrl Pts',(-11.1397779605581,0.177490219299905,6.22305207271077));
#2934=CARTESIAN_POINT('Ctrl Pts',(-11.1965749654798,0.457465808422005,6.2114605744672));
#2935=CARTESIAN_POINT('Ctrl Pts',(-11.2779391678912,0.614760694236416,6.19569689193407));
#2936=CARTESIAN_POINT('Ctrl Pts',(-11.4177773665018,0.822304084339778,6.17123945541837));
#2937=CARTESIAN_POINT('Ctrl Pts',(-11.4776318829417,0.885564567494429,6.16184436313107));
#2938=CARTESIAN_POINT('Ctrl Pts',(-11.6265144893125,1.03369488241838,6.13975499030251));
#2939=CARTESIAN_POINT('Ctrl Pts',(-11.769285484611,1.12926516148223,6.12213126261246));
#2940=CARTESIAN_POINT('Ctrl Pts',(-11.9958937749571,1.22479141349591,6.10347257915889));
#2941=CARTESIAN_POINT('Ctrl Pts',(-12.0734015567445,1.24876937750648,6.09855205886143));
#2942=CARTESIAN_POINT('Ctrl Pts',(-12.2338521859541,1.28348145043716,6.09134419637203));
#2943=CARTESIAN_POINT('Ctrl Pts',(-12.3189795113601,1.2937973652787,6.08913440512663));
#2944=CARTESIAN_POINT('Ctrl Pts',(-12.4739508140748,1.29713192273053,6.08842485041812));
#2945=CARTESIAN_POINT('Ctrl Pts',(-12.5551051454825,1.29286923752959,6.08935069297525));
#2946=CARTESIAN_POINT('Ctrl Pts',(-12.7295007065038,1.26380109840075,6.095447288475));
#2947=CARTESIAN_POINT('Ctrl Pts',(-12.8129106573291,1.2417464539227,6.10003761945498));
#2948=CARTESIAN_POINT('Ctrl Pts',(-12.930645922683,1.19760572832424,6.10879842776981));
#2949=CARTESIAN_POINT('Ctrl Pts',(-12.967672799061,1.18158636714795,6.11192618102656));
#2950=CARTESIAN_POINT('Ctrl Pts',(-13.0777680399706,1.12775712925574,6.12217182297329));
#2951=CARTESIAN_POINT('Ctrl Pts',(-13.1487493610343,1.08425780301533,6.13011818982353));
#2952=CARTESIAN_POINT('Ctrl Pts',(-13.3056808909995,0.96681927406719,6.14991898018366));
#2953=CARTESIAN_POINT('Ctrl Pts',(-13.3666667789338,0.902791579314907,6.15937339329189));
#2954=CARTESIAN_POINT('Ctrl Pts',(-13.4542585130877,0.80419692839569,6.17320967835681));
#2955=CARTESIAN_POINT('Ctrl Pts',(-13.5029326073056,0.737209443905024,6.18166348309254));
#2956=CARTESIAN_POINT('Ctrl Pts',(-13.6075063036529,0.562364326693226,6.20050846236433));
#2957=CARTESIAN_POINT('Ctrl Pts',(-13.6532128199648,0.454665015701439,6.20944139197031));
#2958=CARTESIAN_POINT('Ctrl Pts',(-13.714760512167,0.231511174842811,6.2217703969669));
#2959=CARTESIAN_POINT('Ctrl Pts',(-13.7301962062682,0.116227382741286,6.22506783214625));
#2960=CARTESIAN_POINT('Ctrl Pts',(-13.730193598416,-1.52223171728111E-5,
6.22506754789523));
#2961=CARTESIAN_POINT('Ctrl Pts',(-13.7301935984159,-1.52267580922841E-5,
6.22506754789522));
#2962=CARTESIAN_POINT('Ctrl Pts',(-13.7301907271263,-0.12798100776143,6.22506723488593));
#2963=CARTESIAN_POINT('Ctrl Pts',(-13.7114805449995,-0.254640288623575,
6.22106154775522));
#2964=CARTESIAN_POINT('Ctrl Pts',(-13.6298980591205,-0.521908165468462,
6.2048534383784));
#2965=CARTESIAN_POINT('Ctrl Pts',(-13.5662496906304,-0.638614514310813,
6.19285613210405));
#2966=CARTESIAN_POINT('Ctrl Pts',(-13.4423944644575,-0.823037393434848,
6.17118502256686));
#2967=CARTESIAN_POINT('Ctrl Pts',(-13.3812304072417,-0.886826703639457,
6.16165378610988));
#2968=CARTESIAN_POINT('Ctrl Pts',(-13.2327372610965,-1.0337673323202,6.13975300469276));
#2969=CARTESIAN_POINT('Ctrl Pts',(-13.0886106045117,-1.12971057779523,6.12204728865717));
#2970=CARTESIAN_POINT('Ctrl Pts',(-12.8545066464152,-1.22726329564512,6.1029881561482));
#2971=CARTESIAN_POINT('Ctrl Pts',(-12.7697676836191,-1.25257942206277,6.09777084115763));
#2972=CARTESIAN_POINT('Ctrl Pts',(-12.6009891820413,-1.28598916676046,6.09081125870397));
#2973=CARTESIAN_POINT('Ctrl Pts',(-12.5151371030402,-1.29485665783831,6.08890895085005));
#2974=CARTESIAN_POINT('Ctrl Pts',(-12.4302293937643,-1.29485665783831,6.08890895085005));
#2975=CARTESIAN_POINT('Origin',(-12.4302293937643,0.,0.));
#2976=CARTESIAN_POINT('',(-10.7808324711337,-7.62350904702874E-16,6.22506754791384));
#2977=CARTESIAN_POINT('Origin',(-10.7808324711337,0.,0.));
#2978=CARTESIAN_POINT('',(-12.4302293937643,-7.62350904702875E-16,6.22506754791384));
#2979=CARTESIAN_POINT('',(-14.0796263163949,-7.62350904702874E-16,6.22506754791384));
#2980=CARTESIAN_POINT('',(-12.4302293937643,-7.62350904702875E-16,6.22506754791384));
#2981=CARTESIAN_POINT('Origin',(-14.0796263163949,0.,0.));
#2982=CARTESIAN_POINT('',(-12.4302293937643,6.08890895085005,1.29485665783831));
#2983=CARTESIAN_POINT('Ctrl Pts',(-12.4302293937643,6.08890895085005,1.29485665783831));
#2984=CARTESIAN_POINT('Ctrl Pts',(-12.3718488355339,6.08890895085005,1.29485665783831));
#2985=CARTESIAN_POINT('Ctrl Pts',(-12.3121124409535,6.0897882543227,1.29074255777323));
#2986=CARTESIAN_POINT('Ctrl Pts',(-12.2521561327521,6.09152855044746,1.28247646963738));
#2987=CARTESIAN_POINT('Ctrl Pts',(-12.1926670476362,6.09325528492125,1.27427479686196));
#2988=CARTESIAN_POINT('Ctrl Pts',(-12.1329614629979,6.09582968006873,1.261985531925));
#2989=CARTESIAN_POINT('Ctrl Pts',(-12.0741489521671,6.09918373770257,1.24556160419089));
#2990=CARTESIAN_POINT('Ctrl Pts',(-12.0257014746808,6.10194668098466,1.23203220614457));
#2991=CARTESIAN_POINT('Ctrl Pts',(-11.9778600217895,6.10523781280487,1.21569687634397));
#2992=CARTESIAN_POINT('Ctrl Pts',(-11.9312448343282,6.10899291380237,1.19652478252752));
#2993=CARTESIAN_POINT('Ctrl Pts',(-11.8511268068043,6.11544684655385,1.16357349725477));
#2994=CARTESIAN_POINT('Ctrl Pts',(-11.7746166055436,6.12324782931237,1.12232382755702));
#2995=CARTESIAN_POINT('Ctrl Pts',(-11.7037724666101,6.13154545346576,1.07499596658472));
#2996=CARTESIAN_POINT('Ctrl Pts',(-11.6511399287433,6.13771004271806,1.03983447726073));
#2997=CARTESIAN_POINT('Ctrl Pts',(-11.6016347814191,6.14414724944668,1.00131822095112));
#2998=CARTESIAN_POINT('Ctrl Pts',(-11.556101032204,6.15054104774044,0.960370134973962));
#2999=CARTESIAN_POINT('Ctrl Pts',(-11.5403457122178,6.15275339220543,0.946201519199617));
#3000=CARTESIAN_POINT('Ctrl Pts',(-11.5250658709222,6.1549609506989,0.931741872426695));
#3001=CARTESIAN_POINT('Ctrl Pts',(-11.5102964728551,6.15715212281449,0.917029831909005));
#3002=CARTESIAN_POINT('Ctrl Pts',(-11.4670495554528,6.16356818926938,0.873950865643971));
#3003=CARTESIAN_POINT('Ctrl Pts',(-11.4259525115292,6.17018157540767,0.826420862407318));
#3004=CARTESIAN_POINT('Ctrl Pts',(-11.3879789718363,6.17658890898875,0.775380826076553));
#3005=CARTESIAN_POINT('Ctrl Pts',(-11.3545272206854,6.18223327425541,0.730418502103837));
#3006=CARTESIAN_POINT('Ctrl Pts',(-11.3234993860063,6.18771715669703,0.682732482406092));
#3007=CARTESIAN_POINT('Ctrl Pts',(-11.2955610590574,6.19280256866837,0.632978926651143));
#3008=CARTESIAN_POINT('Ctrl Pts',(-11.2709494590157,6.19728244055603,0.58914972323683));
#3009=CARTESIAN_POINT('Ctrl Pts',(-11.2487354118454,6.20145324377775,0.543716269066643));
#3010=CARTESIAN_POINT('Ctrl Pts',(-11.2293739328148,6.20518515020226,0.497135019687165));
#3011=CARTESIAN_POINT('Ctrl Pts',(-11.2095362147048,6.20900885125039,0.449407999817292));
#3012=CARTESIAN_POINT('Ctrl Pts',(-11.1926931212539,6.21237113545347,0.400470739216812));
#3013=CARTESIAN_POINT('Ctrl Pts',(-11.1788273455236,6.21517025603366,0.350891243271439));
#3014=CARTESIAN_POINT('Ctrl Pts',(-11.1650963685599,6.21794216443263,0.301793743792303));
#3015=CARTESIAN_POINT('Ctrl Pts',(-11.1542851015898,6.22016166015472,0.252066628203633));
#3016=CARTESIAN_POINT('Ctrl Pts',(-11.1463767375417,6.22178063693777,0.202266363778714));
#3017=CARTESIAN_POINT('Ctrl Pts',(-11.1384625687977,6.2234008020409,0.152429546232813));
#3018=CARTESIAN_POINT('Ctrl Pts',(-11.1334555659694,6.22441953396933,0.102519680035822));
#3019=CARTESIAN_POINT('Ctrl Pts',(-11.131338884949,6.22484110271258,0.0530963470502571));
#3020=CARTESIAN_POINT('Ctrl Pts',(-11.130569311005,6.22499437489543,0.0351272204211175));
#3021=CARTESIAN_POINT('Ctrl Pts',(-11.1301818010262,6.22506921164877,0.0172224098454036));
#3022=CARTESIAN_POINT('Ctrl Pts',(-11.1301755454826,6.22506751983931,-0.000591212059548435));
#3023=CARTESIAN_POINT('Ctrl Pts',(-11.1301632788032,6.22506420232037,-0.0355224674101873));
#3024=CARTESIAN_POINT('Ctrl Pts',(-11.131617028533,6.22477123151765,-0.0701045290928973));
#3025=CARTESIAN_POINT('Ctrl Pts',(-11.1345194766772,6.22418013883881,-0.105107446807877));
#3026=CARTESIAN_POINT('Ctrl Pts',(-11.135048849963,6.22407233030683,-0.111491577941726));
#3027=CARTESIAN_POINT('Ctrl Pts',(-11.1356264150422,6.2239544651859,-0.117889707248624));
#3028=CARTESIAN_POINT('Ctrl Pts',(-11.1362520668421,6.22382630456588,-0.124306502983067));
#3029=CARTESIAN_POINT('Ctrl Pts',(-11.1398494021155,6.22308941430334,-0.161201411048983));
#3030=CARTESIAN_POINT('Ctrl Pts',(-11.1450364608977,6.22200768798106,-0.198712719075032));
#3031=CARTESIAN_POINT('Ctrl Pts',(-11.1519002434474,6.2205883070516,-0.236108217271136));
#3032=CARTESIAN_POINT('Ctrl Pts',(-11.1527753381609,6.22040734375055,-0.240875938647017));
#3033=CARTESIAN_POINT('Ctrl Pts',(-11.1536776877754,6.22022096151269,-0.24564177918353));
#3034=CARTESIAN_POINT('Ctrl Pts',(-11.1546074725907,6.22002923635036,-0.250404223280646));
#3035=CARTESIAN_POINT('Ctrl Pts',(-11.1647679800375,6.21793410110223,-0.302447285201551));
#3036=CARTESIAN_POINT('Ctrl Pts',(-11.1782047149051,6.21519654817054,-0.354085778689705));
#3037=CARTESIAN_POINT('Ctrl Pts',(-11.1948269593364,6.21189458999722,-0.404761138022572));
#3038=CARTESIAN_POINT('Ctrl Pts',(-11.2051082660968,6.20985223975804,-0.436105215331061));
#3039=CARTESIAN_POINT('Ctrl Pts',(-11.2166082711959,6.20759503999576,-0.467080908070465));
#3040=CARTESIAN_POINT('Ctrl Pts',(-11.229305507763,6.20515130840228,-0.497557248890469));
#3041=CARTESIAN_POINT('Ctrl Pts',(-11.2511175385676,6.20095332811627,-0.549911230110713));
#3042=CARTESIAN_POINT('Ctrl Pts',(-11.2764626366353,6.19620164677118,-0.600795969759021));
#3043=CARTESIAN_POINT('Ctrl Pts',(-11.3047450780971,6.1910847502828,-0.649565694064773));
#3044=CARTESIAN_POINT('Ctrl Pts',(-11.3362202928213,6.18539021305868,-0.703840978135764));
#3045=CARTESIAN_POINT('Ctrl Pts',(-11.371333470988,6.17924349051508,-0.755496412322283));
#3046=CARTESIAN_POINT('Ctrl Pts',(-11.409263504348,6.17297318268182,-0.803659170283709));
#3047=CARTESIAN_POINT('Ctrl Pts',(-11.4410840719414,6.16771284577818,-0.844064257214491));
#3048=CARTESIAN_POINT('Ctrl Pts',(-11.4748871428235,6.16236744413282,-0.882011602979711));
#3049=CARTESIAN_POINT('Ctrl Pts',(-11.5101879037145,6.15715725915592,-0.916995344652119));
#3050=CARTESIAN_POINT('Ctrl Pts',(-11.5373386303507,6.15314997136772,-0.943902243622234));
#3051=CARTESIAN_POINT('Ctrl Pts',(-11.5659110990122,6.14899975657276,-0.970528187457023));
#3052=CARTESIAN_POINT('Ctrl Pts',(-11.5960932344668,6.14489940158615,-0.995829965644821));
#3053=CARTESIAN_POINT('Ctrl Pts',(-11.5979244007967,6.1446506308521,-0.997365038084425));
#3054=CARTESIAN_POINT('Ctrl Pts',(-11.5997614921715,6.14440205919207,-0.998895239088563));
#3055=CARTESIAN_POINT('Ctrl Pts',(-11.6016045505592,6.14415373553954,-1.00042033673129));
#3056=CARTESIAN_POINT('Ctrl Pts',(-11.6615724669768,6.13607398497985,-1.05004270820941));
#3057=CARTESIAN_POINT('Ctrl Pts',(-11.7278574681358,6.12825826776771,-1.09426801163532));
#3058=CARTESIAN_POINT('Ctrl Pts',(-11.7982730880567,6.12119892536502,-1.13242646216));
#3059=CARTESIAN_POINT('Ctrl Pts',(-11.8606994828957,6.11494052280277,-1.16625552596115));
#3060=CARTESIAN_POINT('Ctrl Pts',(-11.9263723642927,6.10927767330432,-1.19531701975332));
#3061=CARTESIAN_POINT('Ctrl Pts',(-11.993768239231,6.10451864249069,-1.2191464717472));
#3062=CARTESIAN_POINT('Ctrl Pts',(-12.0559835126778,6.10012542994343,-1.24114419598842));
#3063=CARTESIAN_POINT('Ctrl Pts',(-12.1196670734389,6.09650308785304,-1.25868370635078));
#3064=CARTESIAN_POINT('Ctrl Pts',(-12.1836204393827,6.09385116522343,-1.27139449117692));
#3065=CARTESIAN_POINT('Ctrl Pts',(-12.2424548053251,6.09141150963786,-1.28308787048294));
#3066=CARTESIAN_POINT('Ctrl Pts',(-12.3015175131772,6.08979341584715,-1.2906947703834));
#3067=CARTESIAN_POINT('Ctrl Pts',(-12.359875449219,6.08910837609838,-1.29391852920443));
#3068=CARTESIAN_POINT('Ctrl Pts',(-12.3833869081744,6.08883238477606,-1.29521732896233));
#3069=CARTESIAN_POINT('Ctrl Pts',(-12.4067839719209,6.088707294906,-1.29580456658866));
#3070=CARTESIAN_POINT('Ctrl Pts',(-12.4300056202704,6.08873798595888,-1.29566033914429));
#3071=CARTESIAN_POINT('Ctrl Pts',(-12.4891266282453,6.08881612364982,-1.29529314419929));
#3072=CARTESIAN_POINT('Ctrl Pts',(-12.5495196242162,6.08974550575461,-1.29094567075297));
#3073=CARTESIAN_POINT('Ctrl Pts',(-12.6100740656419,6.0915305368075,-1.28246703475439));
#3074=CARTESIAN_POINT('Ctrl Pts',(-12.6686715853072,6.09325788148715,-1.27426240057785));
#3075=CARTESIAN_POINT('Ctrl Pts',(-12.7274202842567,6.09578656737953,-1.26218925802848));
#3076=CARTESIAN_POINT('Ctrl Pts',(-12.7853138452971,6.09907347136525,-1.24610142724366));
#3077=CARTESIAN_POINT('Ctrl Pts',(-12.8340958169417,6.10184306532609,-1.2325455828447));
#3078=CARTESIAN_POINT('Ctrl Pts',(-12.8822706409192,6.10515031552918,-1.21613912550678));
#3079=CARTESIAN_POINT('Ctrl Pts',(-12.9292362816626,6.10894103006689,-1.19678965037943));
#3080=CARTESIAN_POINT('Ctrl Pts',(-13.0093877866196,6.1154102588531,-1.16376785983131));
#3081=CARTESIAN_POINT('Ctrl Pts',(-13.0859056680526,6.12321644231893,-1.12249606627535));
#3082=CARTESIAN_POINT('Ctrl Pts',(-13.1567588548687,6.13151928842058,-1.07514519569055));
#3083=CARTESIAN_POINT('Ctrl Pts',(-13.2098424175907,6.13773982233885,-1.03966968609699));
#3084=CARTESIAN_POINT('Ctrl Pts',(-13.2597463410517,6.1442375291199,-1.00078201446416));
#3085=CARTESIAN_POINT('Ctrl Pts',(-13.3056164890128,6.15069123844581,-0.959407768050671));
#3086=CARTESIAN_POINT('Ctrl Pts',(-13.3209714359044,6.15285160566409,-0.945557815857451));
#3087=CARTESIAN_POINT('Ctrl Pts',(-13.3358743727583,6.15500743188913,-0.931429344163949));
#3088=CARTESIAN_POINT('Ctrl Pts',(-13.3502932603732,6.15714801078641,-0.91705744059957));
#3089=CARTESIAN_POINT('Ctrl Pts',(-13.395064219943,6.16379455480738,-0.872432367528252));
#3090=CARTESIAN_POINT('Ctrl Pts',(-13.4374769917471,6.17063459464968,-0.823155456071043));
#3091=CARTESIAN_POINT('Ctrl Pts',(-13.4764946351208,6.17723981039304,-0.770178096926561));
#3092=CARTESIAN_POINT('Ctrl Pts',(-13.5106703929134,6.18302535339088,-0.723774951116996));
#3093=CARTESIAN_POINT('Ctrl Pts',(-13.5422413743335,6.18863012393773,-0.674532981746127));
#3094=CARTESIAN_POINT('Ctrl Pts',(-13.5705107519144,6.19380382459731,-0.623105254747394));
#3095=CARTESIAN_POINT('Ctrl Pts',(-13.5928556619771,6.19789326291618,-0.5824553348391));
#3096=CARTESIAN_POINT('Ctrl Pts',(-13.6131378073445,6.20171394782517,-0.540440088961139));
#3097=CARTESIAN_POINT('Ctrl Pts',(-13.6310130660832,6.20516488928487,-0.497387849546377));
#3098=CARTESIAN_POINT('Ctrl Pts',(-13.65008358127,6.20884658321043,-0.451456856457475));
#3099=CARTESIAN_POINT('Ctrl Pts',(-13.6664145680264,6.21210579699621,-0.404341033695851));
#3100=CARTESIAN_POINT('Ctrl Pts',(-13.6800047881991,6.21484377769198,-0.356626968937239));
#3101=CARTESIAN_POINT('Ctrl Pts',(-13.693474517426,6.21755748344005,-0.309335937265786));
#3102=CARTESIAN_POINT('Ctrl Pts',(-13.7042518639233,6.21975901285525,-0.261457409881135));
#3103=CARTESIAN_POINT('Ctrl Pts',(-13.7123356221791,6.22140298052968,-0.213567155589214));
#3104=CARTESIAN_POINT('Ctrl Pts',(-13.7204483419628,6.22305283801602,-0.165505325788445));
#3105=CARTESIAN_POINT('Ctrl Pts',(-13.725848138396,6.22414109616072,-0.117431885941534));
#3106=CARTESIAN_POINT('Ctrl Pts',(-13.7285337929633,6.22467474546693,-0.0699306030019548));
#3107=CARTESIAN_POINT('Ctrl Pts',(-13.7298600330228,6.22493827417842,-0.0464733404489176));
#3108=CARTESIAN_POINT('Ctrl Pts',(-13.730524397251,6.22506737084474,-0.0231556133287919));
#3109=CARTESIAN_POINT('Ctrl Pts',(-13.7305267389083,6.22506754773146,-4.7651618804912E-5));
#3110=CARTESIAN_POINT('Ctrl Pts',(-13.7305314774732,6.22506790567845,0.0467134926687206));
#3111=CARTESIAN_POINT('Ctrl Pts',(-13.7278223185331,6.22453713191487,0.0943326037746073));
#3112=CARTESIAN_POINT('Ctrl Pts',(-13.7224017682409,6.22344254907136,0.142228036962457));
#3113=CARTESIAN_POINT('Ctrl Pts',(-13.7169997749408,6.22235171347937,0.189959502447259));
#3114=CARTESIAN_POINT('Ctrl Pts',(-13.7089049231458,6.22070084980274,0.237965202300239));
#3115=CARTESIAN_POINT('Ctrl Pts',(-13.6981196933575,6.2185093699227,0.285669725861333));
#3116=CARTESIAN_POINT('Ctrl Pts',(-13.6872081374435,6.21629222149702,0.333933006886285));
#3117=CARTESIAN_POINT('Ctrl Pts',(-13.673542810278,6.21352173111101,0.381887809531659));
#3118=CARTESIAN_POINT('Ctrl Pts',(-13.6571262805493,6.21027173645692,0.428941645744985));
#3119=CARTESIAN_POINT('Ctrl Pts',(-13.649095512483,6.2086818783252,0.451959814109667));
#3120=CARTESIAN_POINT('Ctrl Pts',(-13.6404063683738,6.2069780829424,0.474762447833064));
#3121=CARTESIAN_POINT('Ctrl Pts',(-13.6310591489254,6.20517347780729,0.49728069176982));
#3122=CARTESIAN_POINT('Ctrl Pts',(-13.60875708102,6.20086776673589,0.551008263713592));
#3123=CARTESIAN_POINT('Ctrl Pts',(-13.5827087264517,6.19598442403786,0.603122184572173));
#3124=CARTESIAN_POINT('Ctrl Pts',(-13.5535786727981,6.1907256556975,0.652979197202176));
#3125=CARTESIAN_POINT('Ctrl Pts',(-13.5210316541874,6.18485003208627,0.708684453953247));
#3126=CARTESIAN_POINT('Ctrl Pts',(-13.4846375656099,6.17850594605293,0.761571903553669));
#3127=CARTESIAN_POINT('Ctrl Pts',(-13.445323369218,6.17204418421574,0.810762951903158));
#3128=CARTESIAN_POINT('Ctrl Pts',(-13.4152322050363,6.16709833884205,0.848413878235033));
#3129=CARTESIAN_POINT('Ctrl Pts',(-13.3834303242871,6.16208535244838,0.883899768089104));
#3130=CARTESIAN_POINT('Ctrl Pts',(-13.3503333798219,6.15718128343761,0.916834019316256));
#3131=CARTESIAN_POINT('Ctrl Pts',(-13.3074383542668,6.15082540470197,0.959518187624141));
#3132=CARTESIAN_POINT('Ctrl Pts',(-13.260254465564,6.14432948438849,1.00006283592689));
#3133=CARTESIAN_POINT('Ctrl Pts',(-13.2096360642912,6.13799486435182,1.03753796136853));
#3134=CARTESIAN_POINT('Ctrl Pts',(-13.1474956494906,6.13021832643703,1.08354336219305));
#3135=CARTESIAN_POINT('Ctrl Pts',(-13.0801792074,6.12268637557024,1.12492259137719));
#3136=CARTESIAN_POINT('Ctrl Pts',(-13.0092673791852,6.11603709544722,1.15998113053774));
#3137=CARTESIAN_POINT('Ctrl Pts',(-12.9830238921301,6.11357628881979,1.17295581109232));
#3138=CARTESIAN_POINT('Ctrl Pts',(-12.9562879674199,6.11123687837181,1.18506500914902));
#3139=CARTESIAN_POINT('Ctrl Pts',(-12.9291397252248,6.10905193800453,1.19622338835736));
#3140=CARTESIAN_POINT('Ctrl Pts',(-12.8721572340207,6.10446588251095,1.21964414026165));
#3141=CARTESIAN_POINT('Ctrl Pts',(-12.8133582604497,6.1005650066165,1.23887411122538));
#3142=CARTESIAN_POINT('Ctrl Pts',(-12.7538653798013,6.09746733340917,1.2539370375334));
#3143=CARTESIAN_POINT('Ctrl Pts',(-12.6943518161327,6.09436858327908,1.26900520054885));
#3144=CARTESIAN_POINT('Ctrl Pts',(-12.6341438628219,6.09207357027527,1.27990354745453));
#3145=CARTESIAN_POINT('Ctrl Pts',(-12.5743652663738,6.09064906637895,1.28664677604512));
#3146=CARTESIAN_POINT('Ctrl Pts',(-12.5258366133329,6.08949264485941,1.2921209728328));
#3147=CARTESIAN_POINT('Ctrl Pts',(-12.4775909192552,6.08890895085005,1.29485665783831));
#3148=CARTESIAN_POINT('Ctrl Pts',(-12.4302293937643,6.08890895085005,1.29485665783831));
#3149=CARTESIAN_POINT('',(-12.4302293937643,-6.08890895085005,-1.29485665783831));
#3150=CARTESIAN_POINT('Ctrl Pts',(-12.4302293937643,-6.08890895085005,-1.29485665783831));
#3151=CARTESIAN_POINT('Ctrl Pts',(-12.3719064521781,-6.08890895085005,-1.29485665783831));
#3152=CARTESIAN_POINT('Ctrl Pts',(-12.3122256701442,-6.08979172951493,-1.29072628612679));
#3153=CARTESIAN_POINT('Ctrl Pts',(-12.2523216952069,-6.09153589587755,-1.28244157969294));
#3154=CARTESIAN_POINT('Ctrl Pts',(-12.1926889042377,-6.09327216643767,-1.27419437794166));
#3155=CARTESIAN_POINT('Ctrl Pts',(-12.1328349365697,-6.09586206915765,-1.261830303888));
#3156=CARTESIAN_POINT('Ctrl Pts',(-12.0738790998279,-6.09923397540106,-1.24531557823849));
#3157=CARTESIAN_POINT('Ctrl Pts',(-12.0255019130074,-6.10200084883197,-1.23176414699457));
#3158=CARTESIAN_POINT('Ctrl Pts',(-11.9777294641826,-6.10529336450592,-1.21541773500516));
#3159=CARTESIAN_POINT('Ctrl Pts',(-11.9311801838106,-6.10904609419394,-1.19625323201392));
#3160=CARTESIAN_POINT('Ctrl Pts',(-11.8510483344045,-6.11550619771905,-1.16326266684596));
#3161=CARTESIAN_POINT('Ctrl Pts',(-11.7745451807163,-6.12331490566863,-1.12196034321072));
#3162=CARTESIAN_POINT('Ctrl Pts',(-11.7036935021763,-6.13161948888405,-1.07457359898116));
#3163=CARTESIAN_POINT('Ctrl Pts',(-11.6511301610919,-6.13778048110204,-1.03941838951899));
#3164=CARTESIAN_POINT('Ctrl Pts',(-11.6016773003432,-6.1442129054961,-1.00091451711278));
#3165=CARTESIAN_POINT('Ctrl Pts',(-11.5561608570514,-6.15060133425726,-0.959983959825811));
#3166=CARTESIAN_POINT('Ctrl Pts',(-11.5403243432848,-6.15282405713949,-0.945743011125359));
#3167=CARTESIAN_POINT('Ctrl Pts',(-11.5249643523102,-6.15504186893641,-0.931208422868594));
#3168=CARTESIAN_POINT('Ctrl Pts',(-11.5101156714317,-6.15724300247758,-0.916419437010658));
#3169=CARTESIAN_POINT('Ctrl Pts',(-11.4645711583886,-6.16399441400674,-0.871058023103533));
#3170=CARTESIAN_POINT('Ctrl Pts',(-11.4214166133875,-6.17094128665832,-0.820917691856838));
#3171=CARTESIAN_POINT('Ctrl Pts',(-11.3817855353081,-6.17764011919321,-0.766960581662782));
#3172=CARTESIAN_POINT('Ctrl Pts',(-11.3472092195376,-6.18348454635098,-0.719885453492252));
#3173=CARTESIAN_POINT('Ctrl Pts',(-11.3153148857571,-6.1891395359759,-0.669905289238284));
#3174=CARTESIAN_POINT('Ctrl Pts',(-11.2868552819188,-6.19434788918216,-0.617673217708659));
#3175=CARTESIAN_POINT('Ctrl Pts',(-11.2655337998714,-6.19824990447424,-0.578541781384198));
#3176=CARTESIAN_POINT('Ctrl Pts',(-11.2461401519929,-6.2019019101112,-0.538146702804389));
#3177=CARTESIAN_POINT('Ctrl Pts',(-11.2289908685175,-6.20521457200396,-0.496767643350301));
#3178=CARTESIAN_POINT('Ctrl Pts',(-11.2095257717429,-6.20897457074771,-0.449800818300852));
#3179=CARTESIAN_POINT('Ctrl Pts',(-11.1929798364322,-6.21228724335781,-0.401664913240023));
#3180=CARTESIAN_POINT('Ctrl Pts',(-11.1793139172197,-6.21505410315874,-0.352942588673756));
#3181=CARTESIAN_POINT('Ctrl Pts',(-11.1658161850305,-6.21778691110363,-0.304819891736394));
#3182=CARTESIAN_POINT('Ctrl Pts',(-11.1551280162058,-6.21998715159152,-0.256125313797636));
#3183=CARTESIAN_POINT('Ctrl Pts',(-11.1472116929566,-6.22161079510395,-0.207424902882935));
#3184=CARTESIAN_POINT('Ctrl Pts',(-11.142675300804,-6.22254121235152,-0.179517482361168));
#3185=CARTESIAN_POINT('Ctrl Pts',(-11.1390491219431,-6.22328324189245,-0.151608217023861));
#3186=CARTESIAN_POINT('Ctrl Pts',(-11.1363260588406,-6.22383632196961,-0.1238039313667));
#3187=CARTESIAN_POINT('Ctrl Pts',(-11.1301829852291,-6.22508403878672,-0.0610790634233799));
#3188=CARTESIAN_POINT('Ctrl Pts',(-11.128636117224,-6.22537741498978,0.00111173707387613));
#3189=CARTESIAN_POINT('Ctrl Pts',(-11.1317392028041,-6.22474640435053,0.0632311443445715));
#3190=CARTESIAN_POINT('Ctrl Pts',(-11.1348422883842,-6.22411539371129,0.125350551615267));
#3191=CARTESIAN_POINT('Ctrl Pts',(-11.1425953275496,-6.22255997486812,0.187398858806157));
#3192=CARTESIAN_POINT('Ctrl Pts',(-11.155052068279,-6.22005198588599,0.249838485757963));
#3193=CARTESIAN_POINT('Ctrl Pts',(-11.1636782663859,-6.21831522261222,0.293077451993458));
#3194=CARTESIAN_POINT('Ctrl Pts',(-11.1745601043725,-6.21611498744589,0.336503678440918));
#3195=CARTESIAN_POINT('Ctrl Pts',(-11.1876619822991,-6.21348992882496,0.379485020100749));
#3196=CARTESIAN_POINT('Ctrl Pts',(-11.2009499746653,-6.21082758079276,0.423076919145163));
#3197=CARTESIAN_POINT('Ctrl Pts',(-11.2165215270484,-6.20772831978472,0.466211022440592));
#3198=CARTESIAN_POINT('Ctrl Pts',(-11.2343395007458,-6.20428609450448,0.508232263466642));
#3199=CARTESIAN_POINT('Ctrl Pts',(-11.2370078547666,-6.20377059954286,0.514525209530911));
#3200=CARTESIAN_POINT('Ctrl Pts',(-11.2397265891724,-6.20324750754818,0.520793208244316));
#3201=CARTESIAN_POINT('Ctrl Pts',(-11.2424955792299,-6.20271723227493,0.527034071507458));
#3202=CARTESIAN_POINT('Ctrl Pts',(-11.2689548168362,-6.19765015757953,0.586668985509251));
#3203=CARTESIAN_POINT('Ctrl Pts',(-11.3000028295008,-6.19192219217637,0.643833523819529));
#3204=CARTESIAN_POINT('Ctrl Pts',(-11.3346739550651,-6.1858270830772,0.697860497777764));
#3205=CARTESIAN_POINT('Ctrl Pts',(-11.3746009810791,-6.17880799801434,0.760077583597297));
#3206=CARTESIAN_POINT('Ctrl Pts',(-11.4193328579437,-6.17130282806334,0.818133275908099));
#3207=CARTESIAN_POINT('Ctrl Pts',(-11.4673948225036,-6.16382680012626,0.871036827083257));
#3208=CARTESIAN_POINT('Ctrl Pts',(-11.4814127796881,-6.1616463099925,0.886466902030723));
#3209=CARTESIAN_POINT('Ctrl Pts',(-11.495714020902,-6.15946861786056,0.901458876654718));
#3210=CARTESIAN_POINT('Ctrl Pts',(-11.5102619553448,-6.15730711289799,0.915988588108959));
#3211=CARTESIAN_POINT('Ctrl Pts',(-11.5532785793428,-6.15091578314529,0.958951328756652));
#3212=CARTESIAN_POINT('Ctrl Pts',(-11.6006222582692,-6.14438414393611,0.99973456931751));
#3213=CARTESIAN_POINT('Ctrl Pts',(-11.6514306134181,-6.13801702466402,1.03740685414387));
#3214=CARTESIAN_POINT('Ctrl Pts',(-11.7142249038981,-6.13014787133441,1.08396621213724));
#3215=CARTESIAN_POINT('Ctrl Pts',(-11.7823113511379,-6.12253156578081,1.12577348439782));
#3216=CARTESIAN_POINT('Ctrl Pts',(-11.8540619600466,-6.1158253205787,1.16109716400415));
#3217=CARTESIAN_POINT('Ctrl Pts',(-11.8793592205985,-6.11346088584032,1.1735513067668));
#3218=CARTESIAN_POINT('Ctrl Pts',(-11.905111962326,-6.11121002907956,1.18519970187327));
#3219=CARTESIAN_POINT('Ctrl Pts',(-11.9312488347654,-6.10910214646688,1.19596694775559));
#3220=CARTESIAN_POINT('Ctrl Pts',(-11.9878698013094,-6.10453578715331,1.21929230431032));
#3221=CARTESIAN_POINT('Ctrl Pts',(-12.0462941969317,-6.10065260800729,1.23844210513609));
#3222=CARTESIAN_POINT('Ctrl Pts',(-12.1054170485769,-6.0975651052557,1.2534615124758));
#3223=CARTESIAN_POINT('Ctrl Pts',(-12.1648706860128,-6.09446032826901,1.26856495173198));
#3224=CARTESIAN_POINT('Ctrl Pts',(-12.2250306169031,-6.09216011743502,1.27949177271444));
#3225=CARTESIAN_POINT('Ctrl Pts',(-12.2847732176283,-6.09072680961869,1.28627870490117));
#3226=CARTESIAN_POINT('Ctrl Pts',(-12.3337654636889,-6.08955141771465,1.29184436571359));
#3227=CARTESIAN_POINT('Ctrl Pts',(-12.3824770589856,-6.08895803534379,1.29462582241761));
#3228=CARTESIAN_POINT('Ctrl Pts',(-12.4302883476924,-6.08895542042789,1.29463812091715));
#3229=CARTESIAN_POINT('Ctrl Pts',(-12.4886595445203,-6.08895222796488,1.29465313574223));
#3230=CARTESIAN_POINT('Ctrl Pts',(-12.5483726894007,-6.08982955021465,1.29054765466148));
#3231=CARTESIAN_POINT('Ctrl Pts',(-12.6083004626829,-6.09156796607547,1.28228923834413));
#3232=CARTESIAN_POINT('Ctrl Pts',(-12.667837119946,-6.0932950362404,1.27408472022353));
#3233=CARTESIAN_POINT('Ctrl Pts',(-12.7275856132271,-6.09587202812029,1.2617812342542));
#3234=CARTESIAN_POINT('Ctrl Pts',(-12.7864405513443,-6.09922962602741,1.24533688015717));
#3235=CARTESIAN_POINT('Ctrl Pts',(-12.8348827488882,-6.10199319058618,1.23180189609072));
#3236=CARTESIAN_POINT('Ctrl Pts',(-12.8827196010596,-6.10528469631702,1.21546142914907));
#3237=CARTESIAN_POINT('Ctrl Pts',(-12.9293347417047,-6.10903936174148,1.19628761290221));
#3238=CARTESIAN_POINT('Ctrl Pts',(-13.0094634914978,-6.1154934159863,1.16332892387194));
#3239=CARTESIAN_POINT('Ctrl Pts',(-13.0859749662094,-6.12329203356386,1.12208290179085));
#3240=CARTESIAN_POINT('Ctrl Pts',(-13.1568259029017,-6.13158884944212,1.07474841590352));
#3241=CARTESIAN_POINT('Ctrl Pts',(-13.2096726789799,-6.13777733461041,1.0394422492776));
#3242=CARTESIAN_POINT('Ctrl Pts',(-13.2593702313246,-6.1442414248502,1.00074886802867));
#3243=CARTESIAN_POINT('Ctrl Pts',(-13.3050706631998,-6.15066229423468,0.959593308839638));
#3244=CARTESIAN_POINT('Ctrl Pts',(-13.320640163871,-6.1528497950107,0.945572182996293));
#3245=CARTESIAN_POINT('Ctrl Pts',(-13.3357457307592,-6.15503267991332,0.931265399040215));
#3246=CARTESIAN_POINT('Ctrl Pts',(-13.3503538359836,-6.15719976089305,0.916709921702932));
#3247=CARTESIAN_POINT('Ctrl Pts',(-13.3951327134421,-6.16384261101928,0.872092366857553));
#3248=CARTESIAN_POINT('Ctrl Pts',(-13.4375529670986,-6.17067969598177,0.822817425220914));
#3249=CARTESIAN_POINT('Ctrl Pts',(-13.4765765828874,-6.17728224695273,0.769837656634619));
#3250=CARTESIAN_POINT('Ctrl Pts',(-13.5107493178741,-6.18306405932469,0.723443606392037));
#3251=CARTESIAN_POINT('Ctrl Pts',(-13.5423173768509,-6.18866540771235,0.674208745551412));
#3252=CARTESIAN_POINT('Ctrl Pts',(-13.5705837162355,-6.19383588730143,0.622786462013254));
#3253=CARTESIAN_POINT('Ctrl Pts',(-13.5929149547238,-6.19792071806891,0.582161347396281));
#3254=CARTESIAN_POINT('Ctrl Pts',(-13.6131854367614,-6.20173719344176,0.540171244993376));
#3255=CARTESIAN_POINT('Ctrl Pts',(-13.6310514543373,-6.20518441878562,0.497144149065676));
#3256=CARTESIAN_POINT('Ctrl Pts',(-13.6501118088316,-6.20886208991722,0.4512407070838));
#3257=CARTESIAN_POINT('Ctrl Pts',(-13.6664354784256,-6.21211785257913,0.404152460898107));
#3258=CARTESIAN_POINT('Ctrl Pts',(-13.6800210197033,-6.21485299465703,0.356466311020465));
#3259=CARTESIAN_POINT('Ctrl Pts',(-13.6934861915508,-6.2175639030672,0.309202665816666));
#3260=CARTESIAN_POINT('Ctrl Pts',(-13.7042615403867,-6.21976323071201,0.26135185013742));
#3261=CARTESIAN_POINT('Ctrl Pts',(-13.7123456608225,-6.22140563057677,0.213489943364428));
#3262=CARTESIAN_POINT('Ctrl Pts',(-13.720459026399,-6.22305397199268,0.165454891200063));
#3263=CARTESIAN_POINT('Ctrl Pts',(-13.7258616567617,-6.22414131346989,0.117408868488908));
#3264=CARTESIAN_POINT('Ctrl Pts',(-13.7285521312143,-6.22467468466975,0.0699360144815334));
#3265=CARTESIAN_POINT('Ctrl Pts',(-13.7298850723235,-6.22493893263467,0.0464165498699207));
#3266=CARTESIAN_POINT('Ctrl Pts',(-13.7305523130127,-6.22506802791389,0.0230377781326179));
#3267=CARTESIAN_POINT('Ctrl Pts',(-13.7305536805202,-6.22506754657021,-0.000129338362996957));
#3268=CARTESIAN_POINT('Ctrl Pts',(-13.7305564396758,-6.22506657538568,-0.04687254071794));
#3269=CARTESIAN_POINT('Ctrl Pts',(-13.7278463221129,-6.22453485270891,-0.0944754434099186));
#3270=CARTESIAN_POINT('Ctrl Pts',(-13.7224257748104,-6.22343961888028,-0.142356194952201));
#3271=CARTESIAN_POINT('Ctrl Pts',(-13.7170239399395,-6.22234816594072,-0.190071655937385));
#3272=CARTESIAN_POINT('Ctrl Pts',(-13.7089303565374,-6.22069701267219,-0.238062851811778));
#3273=CARTESIAN_POINT('Ctrl Pts',(-13.6981474463289,-6.2185054880869,-0.285754213832793));
#3274=CARTESIAN_POINT('Ctrl Pts',(-13.6872385727785,-6.2162883626429,-0.334002694778496));
#3275=CARTESIAN_POINT('Ctrl Pts',(-13.6735771732997,-6.21351817970532,-0.381944090359962));
#3276=CARTESIAN_POINT('Ctrl Pts',(-13.6571657554824,-6.21026868661577,-0.428985799449899));
#3277=CARTESIAN_POINT('Ctrl Pts',(-13.6491280918821,-6.2086772133734,-0.45202496870754));
#3278=CARTESIAN_POINT('Ctrl Pts',(-13.6404307942755,-6.20697158202696,-0.474848405373014));
#3279=CARTESIAN_POINT('Ctrl Pts',(-13.6310741572456,-6.20516495747886,-0.497386998791111));
#3280=CARTESIAN_POINT('Ctrl Pts',(-13.6087805380563,-6.20086039809872,-0.551088645774124));
#3281=CARTESIAN_POINT('Ctrl Pts',(-13.5827438257079,-6.19597875730673,-0.603178538196193));
#3282=CARTESIAN_POINT('Ctrl Pts',(-13.5536276272883,-6.19072206117842,-0.653013275001991));
#3283=CARTESIAN_POINT('Ctrl Pts',(-13.5210961880492,-6.18484877070857,-0.708693473667695));
#3284=CARTESIAN_POINT('Ctrl Pts',(-13.4847204648596,-6.17850748195645,-0.761558070337211));
#3285=CARTESIAN_POINT('Ctrl Pts',(-13.4454260438486,-6.17204874111248,-0.810728261146633));
#3286=CARTESIAN_POINT('Ctrl Pts',(-13.4153072475447,-6.1670981782882,-0.848416740149723));
#3287=CARTESIAN_POINT('Ctrl Pts',(-13.3834736943033,-6.16208041255199,-0.883935191456546));
#3288=CARTESIAN_POINT('Ctrl Pts',(-13.3503421930301,-6.15717216333953,-0.916895265058611));
#3289=CARTESIAN_POINT('Ctrl Pts',(-13.3074631907498,-6.15081987560474,-0.959552404542995));
#3290=CARTESIAN_POINT('Ctrl Pts',(-13.2602991426282,-6.14432752001126,-1.00007419215469));
#3291=CARTESIAN_POINT('Ctrl Pts',(-13.2097032383874,-6.13799606999591,-1.03753082884547));
#3292=CARTESIAN_POINT('Ctrl Pts',(-13.1476353114085,-6.13022903859053,-1.08348031479454));
#3293=CARTESIAN_POINT('Ctrl Pts',(-13.0804028303562,-6.12270564366612,-1.12481689112672));
#3294=CARTESIAN_POINT('Ctrl Pts',(-13.009580870276,-6.11606195335696,-1.15985005875305));
#3295=CARTESIAN_POINT('Ctrl Pts',(-12.9832375841035,-6.11359073348593,-1.17288116886729));
#3296=CARTESIAN_POINT('Ctrl Pts',(-12.9563976650894,-6.11124173558616,-1.18504037709756));
#3297=CARTESIAN_POINT('Ctrl Pts',(-12.9291421733597,-6.1090484410131,-1.19624124717609));
#3298=CARTESIAN_POINT('Ctrl Pts',(-12.8721614715127,-6.10446310953682,-1.21965793856075));
#3299=CARTESIAN_POINT('Ctrl Pts',(-12.8133644404388,-6.10056295946852,-1.2388841534509));
#3300=CARTESIAN_POINT('Ctrl Pts',(-12.7538735725762,-6.09746589322727,-1.2539440406255));
#3301=CARTESIAN_POINT('Ctrl Pts',(-12.694356022634,-6.09436743792968,-1.26901068226714));
#3302=CARTESIAN_POINT('Ctrl Pts',(-12.6341440133822,-6.09207276258628,-1.27990738444859));
#3303=CARTESIAN_POINT('Ctrl Pts',(-12.574361548274,-6.09064854118771,-1.28664926216048));
#3304=CARTESIAN_POINT('Ctrl Pts',(-12.5258340691386,-6.08949245178794,-1.29212187573379));
#3305=CARTESIAN_POINT('Ctrl Pts',(-12.47758962206,-6.08890895085005,-1.29485665783831));
#3306=CARTESIAN_POINT('Ctrl Pts',(-12.4302293937643,-6.08890895085005,-1.29485665783831));
#3307=CARTESIAN_POINT('',(-12.4302293937643,1.29485665783831,-6.08890895085005));
#3308=CARTESIAN_POINT('Ctrl Pts',(-12.4302293937643,1.29485665783831,-6.08890895085005));
#3309=CARTESIAN_POINT('Ctrl Pts',(-12.3719352419111,1.29485665783831,-6.08890895085005));
#3310=CARTESIAN_POINT('Ctrl Pts',(-12.3122852219887,1.29071977209828,-6.08979312075784));
#3311=CARTESIAN_POINT('Ctrl Pts',(-12.2524120064815,1.28242760146153,-6.09153883867612));
#3312=CARTESIAN_POINT('Ctrl Pts',(-12.1927308120721,1.27416202488182,-6.09327895785266));
#3313=CARTESIAN_POINT('Ctrl Pts',(-12.1328278514161,1.26176770689176,-6.09587512987746));
#3314=CARTESIAN_POINT('Ctrl Pts',(-12.0738249340326,1.24521625255819,-6.09925425445234));
#3315=CARTESIAN_POINT('Ctrl Pts',(-12.0254691329447,1.23165151933884,-6.10202361371524));
#3316=CARTESIAN_POINT('Ctrl Pts',(-11.9777178559071,1.21529437282654,-6.10531793806464));
#3317=CARTESIAN_POINT('Ctrl Pts',(-11.9311886135114,1.19612476042382,-6.10907124967381));
#3318=CARTESIAN_POINT('Ctrl Pts',(-11.8510584764837,1.16311189390145,-6.11553499930876));
#3319=CARTESIAN_POINT('Ctrl Pts',(-11.7745547714117,1.12179911546558,-6.12334463259387));
#3320=CARTESIAN_POINT('Ctrl Pts',(-11.703704178694,1.07438858878809,-6.13165190926328));
#3321=CARTESIAN_POINT('Ctrl Pts',(-11.6508998934495,1.03905396591142,-6.13784324500275));
#3322=CARTESIAN_POINT('Ctrl Pts',(-11.6012356756643,1.00033238611109,-6.14430943936365));
#3323=CARTESIAN_POINT('Ctrl Pts',(-11.5555505260111,0.959148077021043,-6.15073174040592));
#3324=CARTESIAN_POINT('Ctrl Pts',(-11.5399372428507,0.945072993882056,-6.15292661566572));
#3325=CARTESIAN_POINT('Ctrl Pts',(-11.52478871006,0.930710387099588,-6.15511676685479));
#3326=CARTESIAN_POINT('Ctrl Pts',(-11.5101384180024,0.916097539649635,-6.15729090379348));
#3327=CARTESIAN_POINT('Ctrl Pts',(-11.4598732878207,0.865960881860794,-6.16475036438488));
#3328=CARTESIAN_POINT('Ctrl Pts',(-11.4124955062379,0.81018432415652,-6.17241979163684));
#3329=CARTESIAN_POINT('Ctrl Pts',(-11.3695630860768,0.749809784999349,-6.17974524251682));
#3330=CARTESIAN_POINT('Ctrl Pts',(-11.3330563251016,0.698471452295889,-6.18597429933));
#3331=CARTESIAN_POINT('Ctrl Pts',(-11.2997638384491,0.643808791677128,-6.19195383145789));
#3332=CARTESIAN_POINT('Ctrl Pts',(-11.2706435584294,0.586479899545217,-6.1973790672767));
#3333=CARTESIAN_POINT('Ctrl Pts',(-11.2556374283266,0.556937435894595,-6.20017477509545));
#3334=CARTESIAN_POINT('Ctrl Pts',(-11.2417392277346,0.52668723531776,-6.20282398036088));
#3335=CARTESIAN_POINT('Ctrl Pts',(-11.2290800420475,0.495821129429846,-6.20529027392764));
#3336=CARTESIAN_POINT('Ctrl Pts',(-11.1986034220322,0.421511880498185,-6.21122780369755));
#3337=CARTESIAN_POINT('Ctrl Pts',(-11.1751084916239,0.34613055315122,-6.21590342372622));
#3338=CARTESIAN_POINT('Ctrl Pts',(-11.1586345171804,0.270072365609977,-6.21920629127414));
#3339=CARTESIAN_POINT('Ctrl Pts',(-11.1422659320947,0.194500746963393,-6.2224880293071));
#3340=CARTESIAN_POINT('Ctrl Pts',(-11.1328287596466,0.118261199967257,-6.22441440835855));
#3341=CARTESIAN_POINT('Ctrl Pts',(-11.1303615174059,0.0417484625205447,
-6.22492755315009));
#3342=CARTESIAN_POINT('Ctrl Pts',(-11.1279029777771,-0.0344943943881157,
-6.22543888794507));
#3343=CARTESIAN_POINT('Ctrl Pts',(-11.1323652855205,-0.111008206921567,
-6.22454690271329));
#3344=CARTESIAN_POINT('Ctrl Pts',(-11.1437865520568,-0.187399937894528,
-6.22224615708565));
#3345=CARTESIAN_POINT('Ctrl Pts',(-11.1469051234995,-0.208258664018226,
-6.22161793957682));
#3346=CARTESIAN_POINT('Ctrl Pts',(-11.1505425273872,-0.2291082890747,-6.22088499036746));
#3347=CARTESIAN_POINT('Ctrl Pts',(-11.1546995395729,-0.249940827291389,
-6.22004787432886));
#3348=CARTESIAN_POINT('Ctrl Pts',(-11.1642432734415,-0.297768495738485,
-6.21812601017916));
#3349=CARTESIAN_POINT('Ctrl Pts',(-11.1765257430138,-0.345509865059888,
-6.21565068788586));
#3350=CARTESIAN_POINT('Ctrl Pts',(-11.1914688466414,-0.392581270096085,
-6.21267622868436));
#3351=CARTESIAN_POINT('Ctrl Pts',(-11.2067889055284,-0.440840100056904,
-6.20962673567008));
#3352=CARTESIAN_POINT('Ctrl Pts',(-11.2249055260701,-0.488394527974946,
-6.20605265433493));
#3353=CARTESIAN_POINT('Ctrl Pts',(-11.2457345456789,-0.534621239870226,
-6.20206788950022));
#3354=CARTESIAN_POINT('Ctrl Pts',(-11.2578471921851,-0.561503341421173,
-6.19975063939629));
#3355=CARTESIAN_POINT('Ctrl Pts',(-11.2708771019852,-0.587936568342572,
-6.19729554156883));
#3356=CARTESIAN_POINT('Ctrl Pts',(-11.2848077238703,-0.613799570314091,
-6.19473292915621));
#3357=CARTESIAN_POINT('Ctrl Pts',(-11.317012279437,-0.673589182793906,-6.18880872889301));
#3358=CARTESIAN_POINT('Ctrl Pts',(-11.3540305414379,-0.730333687517002,
-6.18230771173298));
#3359=CARTESIAN_POINT('Ctrl Pts',(-11.3943190776739,-0.783294411432698,
-6.17559032328962));
#3360=CARTESIAN_POINT('Ctrl Pts',(-11.4306575667326,-0.831062656853222,
-6.16953153413375));
#3361=CARTESIAN_POINT('Ctrl Pts',(-11.469656504718,-0.87575311065843,-6.16329845093917));
#3362=CARTESIAN_POINT('Ctrl Pts',(-11.5101833773516,-0.916837225683864,
-6.15718080599314));
#3363=CARTESIAN_POINT('Ctrl Pts',(-11.5648237040178,-0.972228854001241,
-6.14893269562692));
#3364=CARTESIAN_POINT('Ctrl Pts',(-11.6274857929233,-1.02318325634266,-6.14057642072509));
#3365=CARTESIAN_POINT('Ctrl Pts',(-11.6956087254554,-1.06850889312374,-6.13267924494715));
#3366=CARTESIAN_POINT('Ctrl Pts',(-11.7680959781152,-1.1167383330964,-6.12427613376803));
#3367=CARTESIAN_POINT('Ctrl Pts',(-11.8467661895401,-1.15859576110227,-6.11639821025487));
#3368=CARTESIAN_POINT('Ctrl Pts',(-11.9285340363439,-1.19266902583605,-6.10974684998498));
#3369=CARTESIAN_POINT('Ctrl Pts',(-11.9925136718482,-1.21932981174788,-6.10454246192402));
#3370=CARTESIAN_POINT('Ctrl Pts',(-12.0583897892245,-1.24122576538538,-6.10009072445943));
#3371=CARTESIAN_POINT('Ctrl Pts',(-12.124684375347,-1.2576802310512,-6.09669635232993));
#3372=CARTESIAN_POINT('Ctrl Pts',(-12.143116210675,-1.26225505411446,-6.09575261752755));
#3373=CARTESIAN_POINT('Ctrl Pts',(-12.161580393752,-1.26640921081734,-6.09489032856723));
#3374=CARTESIAN_POINT('Ctrl Pts',(-12.1800451595059,-1.27012803811809,-6.09411525513559));
#3375=CARTESIAN_POINT('Ctrl Pts',(-12.2370752874949,-1.28161397840879,-6.09172136952683));
#3376=CARTESIAN_POINT('Ctrl Pts',(-12.2941109738721,-1.28894330191908,-6.09016446666203));
#3377=CARTESIAN_POINT('Ctrl Pts',(-12.3512598524599,-1.29234468050352,-6.08944260198454));
#3378=CARTESIAN_POINT('Ctrl Pts',(-12.4111984809399,-1.2959120990134,-6.08868549913693));
#3379=CARTESIAN_POINT('Ctrl Pts',(-12.4712616224261,-1.29515870258049,-6.08884670582411));
#3380=CARTESIAN_POINT('Ctrl Pts',(-12.5315734553096,-1.2903366772538,-6.08986840871161));
#3381=CARTESIAN_POINT('Ctrl Pts',(-12.5395566571344,-1.28969840778749,-6.09000364685586));
#3382=CARTESIAN_POINT('Ctrl Pts',(-12.5475442161835,-1.28898883805471,-6.09015388866053));
#3383=CARTESIAN_POINT('Ctrl Pts',(-12.555536420442,-1.28820853927745,-6.09031893544359));
#3384=CARTESIAN_POINT('Ctrl Pts',(-12.6148621992992,-1.28241641595264,-6.09154407041708));
#3385=CARTESIAN_POINT('Ctrl Pts',(-12.6744439304571,-1.27272832674441,-6.09358899140211));
#3386=CARTESIAN_POINT('Ctrl Pts',(-12.7334612362498,-1.25894040366121,-6.09643625703733));
#3387=CARTESIAN_POINT('Ctrl Pts',(-12.7903656500025,-1.24564610516046,-6.09918158706545));
#3388=CARTESIAN_POINT('Ctrl Pts',(-12.846745329193,-1.22854021111248,-6.10267301592439));
#3389=CARTESIAN_POINT('Ctrl Pts',(-12.9018648908817,-1.20743110787297,-6.10684665730446));
#3390=CARTESIAN_POINT('Ctrl Pts',(-12.9109361860556,-1.20395707976975,-6.10753353382795));
#3391=CARTESIAN_POINT('Ctrl Pts',(-12.9199733510849,-1.20037460654414,-6.10823877499836));
#3392=CARTESIAN_POINT('Ctrl Pts',(-12.9289731080053,-1.19668281244561,-6.1089619594893));
#3393=CARTESIAN_POINT('Ctrl Pts',(-13.0092397676277,-1.16375659200186,-6.11541186740248));
#3394=CARTESIAN_POINT('Ctrl Pts',(-13.0857840883755,-1.12253184392904,-6.12320982866879));
#3395=CARTESIAN_POINT('Ctrl Pts',(-13.1566294645525,-1.07518791339112,-6.13151179783483));
#3396=CARTESIAN_POINT('Ctrl Pts',(-13.2097039744373,-1.03971974249676,-6.13773129963358));
#3397=CARTESIAN_POINT('Ctrl Pts',(-13.2595800061123,-1.00081730251846,-6.14423201250788));
#3398=CARTESIAN_POINT('Ctrl Pts',(-13.305426478321,-0.959409544350473,-6.15069096137168));
#3399=CARTESIAN_POINT('Ctrl Pts',(-13.3207771905434,-0.945545040741119,
-6.15285360247559));
#3400=CARTESIAN_POINT('Ctrl Pts',(-13.3356761479583,-0.93139978266754,-6.15501195034366));
#3401=CARTESIAN_POINT('Ctrl Pts',(-13.3500921536751,-0.917009010794008,
-6.1571552238199));
#3402=CARTESIAN_POINT('Ctrl Pts',(-13.3976333039604,-0.869551076758588,
-6.16422331802285));
#3403=CARTESIAN_POINT('Ctrl Pts',(-13.4425608636519,-0.81703406747505,-6.17148062215402));
#3404=CARTESIAN_POINT('Ctrl Pts',(-13.483600558711,-0.760436921636467,-6.17844654134857));
#3405=CARTESIAN_POINT('Ctrl Pts',(-13.5191371378058,-0.711429029478902,
-6.18447838291243));
#3406=CARTESIAN_POINT('Ctrl Pts',(-13.5517586124413,-0.659362108365003,
-6.1902910582668));
#3407=CARTESIAN_POINT('Ctrl Pts',(-13.5806376553944,-0.604887217003585,
-6.19560952859327));
#3408=CARTESIAN_POINT('Ctrl Pts',(-13.599039804785,-0.570175017901222,-6.19899853582721));
#3409=CARTESIAN_POINT('Ctrl Pts',(-13.6159223677976,-0.534485392014676,
-6.20218766535699));
#3410=CARTESIAN_POINT('Ctrl Pts',(-13.6310712848955,-0.497989969556114,
-6.20511659570644));
#3411=CARTESIAN_POINT('Ctrl Pts',(-13.6491844766246,-0.454353280547129,
-6.2086186464892));
#3412=CARTESIAN_POINT('Ctrl Pts',(-13.6648191782393,-0.409558830596979,
-6.21174609228389));
#3413=CARTESIAN_POINT('Ctrl Pts',(-13.677970884626,-0.364227652922393,-6.21440296351441));
#3414=CARTESIAN_POINT('Ctrl Pts',(-13.6909855338216,-0.319368882682671,
-6.21703214683151));
#3415=CARTESIAN_POINT('Ctrl Pts',(-13.7015686699469,-0.273984691860296,
-6.21920039368607));
#3416=CARTESIAN_POINT('Ctrl Pts',(-13.709715927272,-0.228681285226899,-6.22086576337064));
#3417=CARTESIAN_POINT('Ctrl Pts',(-13.715963806497,-0.193939506265998,-6.2221428837854));
#3418=CARTESIAN_POINT('Ctrl Pts',(-13.7207791744087,-0.159245349452789,
-6.22312532680939));
#3419=CARTESIAN_POINT('Ctrl Pts',(-13.7241600621217,-0.124872935992544,
-6.22381496559358));
#3420=CARTESIAN_POINT('Ctrl Pts',(-13.7279291532591,-0.0865537813983614,
-6.2245837907218));
#3421=CARTESIAN_POINT('Ctrl Pts',(-13.7299154291426,-0.0486342986908554,
-6.22499491309192));
#3422=CARTESIAN_POINT('Ctrl Pts',(-13.7301623651014,-0.0104114932913323,
-6.22505884123977));
#3423=CARTESIAN_POINT('Ctrl Pts',(-13.730182837164,-0.0072426568496272,
-6.22506414116066));
#3424=CARTESIAN_POINT('Ctrl Pts',(-13.7301913545179,-0.00407173538213392,
-6.22506702514711));
#3425=CARTESIAN_POINT('Ctrl Pts',(-13.7301879419361,-0.000898328273157036,
-6.22506748309577));
#3426=CARTESIAN_POINT('Ctrl Pts',(-13.7301342273928,0.0490515694210033,
-6.22507469127552));
#3427=CARTESIAN_POINT('Ctrl Pts',(-13.7271248442808,0.0996193688592282,
-6.22447648964631));
#3428=CARTESIAN_POINT('Ctrl Pts',(-13.7211337179369,0.150256489319034,-6.22325388872313));
#3429=CARTESIAN_POINT('Ctrl Pts',(-13.715142788269,0.200891947469772,-6.22203132793534));
#3430=CARTESIAN_POINT('Ctrl Pts',(-13.7061703111347,0.251596510611804,-6.22018438455461));
#3431=CARTESIAN_POINT('Ctrl Pts',(-13.6941902144386,0.301822616132018,-6.21774630267923));
#3432=CARTESIAN_POINT('Ctrl Pts',(-13.6820411900285,0.35275694474944,-6.21527384214999));
#3433=CARTESIAN_POINT('Ctrl Pts',(-13.6667991289883,0.403199012571096,-6.21219350738699));
#3434=CARTESIAN_POINT('Ctrl Pts',(-13.6484368406936,0.452582026989457,-6.20859368012887));
#3435=CARTESIAN_POINT('Ctrl Pts',(-13.6429068058991,0.467454344840342,-6.20750954673156));
#3436=CARTESIAN_POINT('Ctrl Pts',(-13.6370937698569,0.482230648591652,-6.20637865560157));
#3437=CARTESIAN_POINT('Ctrl Pts',(-13.6309969898517,0.496895573243171,-6.20520432905971));
#3438=CARTESIAN_POINT('Ctrl Pts',(-13.6095308024466,0.548529389877824,-6.2010696360577));
#3439=CARTESIAN_POINT('Ctrl Pts',(-13.5845471044433,0.598788311474538,-6.19639176855541));
#3440=CARTESIAN_POINT('Ctrl Pts',(-13.5566725551178,0.647027314399991,-6.19135054980013));
#3441=CARTESIAN_POINT('Ctrl Pts',(-13.5257682528023,0.700509532619786,-6.1857613886398));
#3442=CARTESIAN_POINT('Ctrl Pts',(-13.4913105190966,0.7515085229059,-6.17972570509742));
#3443=CARTESIAN_POINT('Ctrl Pts',(-13.4541533675084,0.799161663499016,-6.17355704692874));
#3444=CARTESIAN_POINT('Ctrl Pts',(-13.421364771179,0.841212238528311,-6.16811363606592));
#3445=CARTESIAN_POINT('Ctrl Pts',(-13.3864741834141,0.880657802541923,-6.1625685925932));
#3446=CARTESIAN_POINT('Ctrl Pts',(-13.3500684256529,0.916916483466317,-6.15716900356307));
#3447=CARTESIAN_POINT('Ctrl Pts',(-13.3072843024532,0.959527761657628,-6.1508233951621));
#3448=CARTESIAN_POINT('Ctrl Pts',(-13.2602024392506,1.000011743866,-6.14433750063204));
#3449=CARTESIAN_POINT('Ctrl Pts',(-13.2096808645379,1.03743921852613,-6.13801155456341));
#3450=CARTESIAN_POINT('Ctrl Pts',(-13.1477978650733,1.08328348223975,-6.13026301308574));
#3451=CARTESIAN_POINT('Ctrl Pts',(-13.0807541375615,1.12454175109865,-6.12275592889658));
#3452=CARTESIAN_POINT('Ctrl Pts',(-13.0101265129726,1.15953221587873,-6.11612222052743));
#3453=CARTESIAN_POINT('Ctrl Pts',(-12.9835946088692,1.17267669952065,-6.11363020815516));
#3454=CARTESIAN_POINT('Ctrl Pts',(-12.9565569462931,1.18493690018302,-6.11126196523134));
#3455=CARTESIAN_POINT('Ctrl Pts',(-12.9290971176065,1.19622424046656,-6.10905177115158));
#3456=CARTESIAN_POINT('Ctrl Pts',(-12.8721127877878,1.21964760296576,-6.10446520108074));
#3457=CARTESIAN_POINT('Ctrl Pts',(-12.8133104381631,1.23887976609541,-6.10056386132526));
#3458=CARTESIAN_POINT('Ctrl Pts',(-12.75381277262,1.25394388410792,-6.09746592541511));
#3459=CARTESIAN_POINT('Ctrl Pts',(-12.694302849074,1.2690111057044,-6.09436735125291));
#3460=CARTESIAN_POINT('Ctrl Pts',(-12.6340973230754,1.27990869110762,-6.09207248827396));
#3461=CARTESIAN_POINT('Ctrl Pts',(-12.5743195925698,1.28665074919624,-6.09064822705127));
#3462=CARTESIAN_POINT('Ctrl Pts',(-12.5258076391736,1.29212219157157,-6.08949238367156));
#3463=CARTESIAN_POINT('Ctrl Pts',(-12.4775774299124,1.29485665783831,-6.08890895085005));
#3464=CARTESIAN_POINT('Ctrl Pts',(-12.4302293937643,1.29485665783831,-6.08890895085005));
#3465=CARTESIAN_POINT('Origin',(-12.4302293937643,0.,0.));
#3466=CARTESIAN_POINT('',(-13.4302293937643,9.49101269339199E-16,4.5));
#3467=CARTESIAN_POINT('Origin',(-12.4302293937643,8.26636589424463E-16,
4.5));
#3468=CARTESIAN_POINT('',(-13.4302293937643,-1.22464679914735E-16,2.24963967399279E-32));
#3469=CARTESIAN_POINT('Ctrl Pts',(-12.4302293937643,6.08898133099087,1.29494387859312));
#3470=CARTESIAN_POINT('Ctrl Pts',(-12.5942619533871,6.08898130876529,1.29494384540356));
#3471=CARTESIAN_POINT('Ctrl Pts',(-12.9435374583722,6.10366925625812,1.22945303091367));
#3472=CARTESIAN_POINT('Ctrl Pts',(-13.2353404857064,6.14038646272546,1.03141337526286));
#3473=CARTESIAN_POINT('Ctrl Pts',(-13.4654395118979,6.17439967538392,0.802430842761209));
#3474=CARTESIAN_POINT('Ctrl Pts',(-13.6642427239162,6.21076528208221,0.511664182013643));
#3475=CARTESIAN_POINT('Ctrl Pts',(-13.7306321021329,6.22545881283488,0.163545778636827));
#3476=CARTESIAN_POINT('Ctrl Pts',(-13.7305989411604,6.22543847090119,-0.163641090648478));
#3477=CARTESIAN_POINT('Ctrl Pts',(-13.6642156833053,6.21072435088059,-0.511783667678438));
#3478=CARTESIAN_POINT('Ctrl Pts',(-13.4653424297833,6.17435111576691,-0.802515858885917));
#3479=CARTESIAN_POINT('Ctrl Pts',(-13.2353573393715,6.1402285928138,-1.03175436379926));
#3480=CARTESIAN_POINT('Ctrl Pts',(-13.0895788709221,6.12205139295494,-1.13084360876944));
#3481=CARTESIAN_POINT('Ctrl Pts',(-12.7689529244921,6.09609767279734,-1.26292405472951));
#3482=CARTESIAN_POINT('Ctrl Pts',(-12.5945528226149,6.08914675284976,-1.29475090526595));
#3483=CARTESIAN_POINT('Ctrl Pts',(-12.1420480242785,6.08829833850425,-1.29750804265229));
#3484=CARTESIAN_POINT('Ctrl Pts',(-11.7821275442938,6.1174178096963,-1.17136422515573));
#3485=CARTESIAN_POINT('Ctrl Pts',(-11.5389300175645,6.15310688833719,-0.945622018154235));
#3486=CARTESIAN_POINT('Ctrl Pts',(-11.3949322424527,6.17435262252434,-0.802915209412389));
#3487=CARTESIAN_POINT('Ctrl Pts',(-11.2460566890049,6.20152475294844,-0.584204969074392));
#3488=CARTESIAN_POINT('Ctrl Pts',(-11.1584525181573,6.21935644205315,-0.293078203033809));
#3489=CARTESIAN_POINT('Ctrl Pts',(-11.1341427705081,6.22436148348913,-0.123532917714704));
#3490=CARTESIAN_POINT('Ctrl Pts',(-11.1219312944025,6.22705283541575,0.121373316802368));
#3491=CARTESIAN_POINT('Ctrl Pts',(-11.195852637914,6.21080281923344,0.510717187316461));
#3492=CARTESIAN_POINT('Ctrl Pts',(-11.3953251934327,6.17426182590549,0.802628398668338));
#3493=CARTESIAN_POINT('Ctrl Pts',(-11.6251545032248,6.14020379361964,1.03156839761272));
#3494=CARTESIAN_POINT('Ctrl Pts',(-11.7709691894469,6.12201232016596,1.13070854621628));
#3495=CARTESIAN_POINT('Ctrl Pts',(-12.0914612527931,6.09613472840634,1.26250865035172));
#3496=CARTESIAN_POINT('Ctrl Pts',(-12.2661968588882,6.08898130665445,1.29494390504147));
#3497=CARTESIAN_POINT('Ctrl Pts',(-12.4302293937643,6.08898133099087,1.29494387859312));
#3498=CARTESIAN_POINT('Ctrl Pts',(-12.4302293937643,6.00722696133003,1.19642683026457));
#3499=CARTESIAN_POINT('Ctrl Pts',(-12.5835311917541,6.00725206547108,1.19646431839136));
#3500=CARTESIAN_POINT('Ctrl Pts',(-12.909964007985,6.02008795273409,1.13389253469307));
#3501=CARTESIAN_POINT('Ctrl Pts',(-13.1794216562216,6.05199550620319,0.947617208560084));
#3502=CARTESIAN_POINT('Ctrl Pts',(-13.3904648409007,6.08141552880984,0.734503844042364));
#3503=CARTESIAN_POINT('Ctrl Pts',(-13.570887885006,6.11264821229161,0.465895827821163));
#3504=CARTESIAN_POINT('Ctrl Pts',(-13.63034543552,6.12520612798745,0.148902652084511));
#3505=CARTESIAN_POINT('Ctrl Pts',(-13.6303230222317,6.12518235248142,-0.148993075746921));
#3506=CARTESIAN_POINT('Ctrl Pts',(-13.570842515833,6.11261315450347,-0.466033199953071));
#3507=CARTESIAN_POINT('Ctrl Pts',(-13.3903856984601,6.08136116262512,-0.734565587427399));
#3508=CARTESIAN_POINT('Ctrl Pts',(-13.179410253184,6.05184812885104,-0.948000402118588));
#3509=CARTESIAN_POINT('Ctrl Pts',(-13.044873465078,6.03604579828012,-1.04111526370645));
#3510=CARTESIAN_POINT('Ctrl Pts',(-12.7467548427922,6.01347833294355,-1.16594234995302));
#3511=CARTESIAN_POINT('Ctrl Pts',(-12.5838837655095,6.00734418127635,-1.19625532919237));
#3512=CARTESIAN_POINT('Ctrl Pts',(-12.1607096950123,6.00667035326614,-1.19893255050596));
#3513=CARTESIAN_POINT('Ctrl Pts',(-11.8251276746147,6.03213208496433,-1.07836492136828));
#3514=CARTESIAN_POINT('Ctrl Pts',(-11.6020268212092,6.06296598113213,-0.867855162821189));
#3515=CARTESIAN_POINT('Ctrl Pts',(-11.4699415156986,6.08136857971696,-0.734854564014157));
#3516=CARTESIAN_POINT('Ctrl Pts',(-11.3347377808286,6.10471391255857,-0.533003961090166));
#3517=CARTESIAN_POINT('Ctrl Pts',(-11.2558516212822,6.11997308110787,-0.266984478934218));
#3518=CARTESIAN_POINT('Ctrl Pts',(-11.2339578831136,6.1242543025212,-0.112499763704596));
#3519=CARTESIAN_POINT('Ctrl Pts',(-11.2230782222799,6.12653186075723,0.110502918514062));
#3520=CARTESIAN_POINT('Ctrl Pts',(-11.2892260889657,6.11268306432087,0.465058908284595));
#3521=CARTESIAN_POINT('Ctrl Pts',(-11.4702873307785,6.08127779974347,0.734631343754487));
#3522=CARTESIAN_POINT('Ctrl Pts',(-11.681094900266,6.05181289859711,0.947846902939449));
#3523=CARTESIAN_POINT('Ctrl Pts',(-11.8156864487299,6.03603021308043,1.04095287446958));
#3524=CARTESIAN_POINT('Ctrl Pts',(-12.1136410603724,6.01347722311489,1.16555887365695));
#3525=CARTESIAN_POINT('Ctrl Pts',(-12.2768996439547,6.0072544496917,1.19639695643086));
#3526=CARTESIAN_POINT('Ctrl Pts',(-12.4302293937643,6.00722696133003,1.19642683026457));
#3527=CARTESIAN_POINT('Ctrl Pts',(-12.4302293937643,5.9254725916692,1.09790978193603));
#3528=CARTESIAN_POINT('Ctrl Pts',(-12.5728345397284,5.92544735481571,1.09787209562915));
#3529=CARTESIAN_POINT('Ctrl Pts',(-12.8763450487991,5.93647960612607,1.03842675040526));
#3530=CARTESIAN_POINT('Ctrl Pts',(-13.1235630570658,5.96359104894073,0.863676007684786));
#3531=CARTESIAN_POINT('Ctrl Pts',(-13.3154843928422,5.98836813882517,0.666454964337181));
#3532=CARTESIAN_POINT('Ctrl Pts',(-13.4776843866789,6.0145609350393,0.420230715694402));
#3533=CARTESIAN_POINT('Ctrl Pts',(-13.5299505040167,6.0248593589734,0.134217204930517));
#3534=CARTESIAN_POINT('Ctrl Pts',(-13.5299007211169,6.02484699389389,-0.134415017109032));
#3535=CARTESIAN_POINT('Ctrl Pts',(-13.4776660945839,6.01452487292353,-0.420420663484723));
#3536=CARTESIAN_POINT('Ctrl Pts',(-13.3153544274694,5.98833547677297,-0.666673705537073));
#3537=CARTESIAN_POINT('Ctrl Pts',(-13.1235774765046,5.96346920539124,-0.864075760813053));
#3538=CARTESIAN_POINT('Ctrl Pts',(-13.0001273339958,5.9500823476246,-0.951353330164833));
#3539=CARTESIAN_POINT('Ctrl Pts',(-12.7246790600745,5.93077700575973,-1.06883672236603));
#3540=CARTESIAN_POINT('Ctrl Pts',(-12.5731730637106,5.92562762457043,-1.09763635624804));
#3541=CARTESIAN_POINT('Ctrl Pts',(-12.1795045349912,5.92492523315675,-1.10023761151678));
#3542=CARTESIAN_POINT('Ctrl Pts',(-11.8682715322971,5.94673197605431,-0.98542923697083));
#3543=CARTESIAN_POINT('Ctrl Pts',(-11.6651441685123,5.97286503936011,-0.789835019063647));
#3544=CARTESIAN_POINT('Ctrl Pts',(-11.5449751521618,5.98831895514578,-0.667076440523771));
#3545=CARTESIAN_POINT('Ctrl Pts',(-11.4234880389121,6.00790204058972,-0.48164167101503));
#3546=CARTESIAN_POINT('Ctrl Pts',(-11.3532980958741,6.02055638021736,-0.240902614043722));
#3547=CARTESIAN_POINT('Ctrl Pts',(-11.3338748805631,6.0241045391149,-0.101410210808414));
#3548=CARTESIAN_POINT('Ctrl Pts',(-11.324192538491,6.02601447481949,0.0996219915262307));
#3549=CARTESIAN_POINT('Ctrl Pts',(-11.3825655879323,6.01457216711308,0.419448146088014));
#3550=CARTESIAN_POINT('Ctrl Pts',(-11.5452549217081,5.98827602700875,0.666788336702704));
#3551=CARTESIAN_POINT('Ctrl Pts',(-11.7369439829688,5.96346321923707,0.863887776934397));
#3552=CARTESIAN_POINT('Ctrl Pts',(-11.8604202279154,5.95003321189189,0.951280997109748));
#3553=CARTESIAN_POINT('Ctrl Pts',(-12.1357679453513,5.93083589668504,1.06847119991178));
#3554=CARTESIAN_POINT('Ctrl Pts',(-12.2876523473866,5.92544495799094,1.09793981369705));
#3555=CARTESIAN_POINT('Ctrl Pts',(-12.4302293937643,5.9254725916692,1.09790978193603));
#3556=CARTESIAN_POINT('Ctrl Pts',(-12.4302293937643,5.84371822200836,0.999392733607483));
#3557=CARTESIAN_POINT('Ctrl Pts',(-12.5621036578468,5.84371837757123,0.99939296591021));
#3558=CARTESIAN_POINT('Ctrl Pts',(-12.8427717588467,5.8528983979387,0.942865920290856));
#3559=CARTESIAN_POINT('Ctrl Pts',(-13.0676440152473,5.87520014001345,0.779880352279897));
#3560=CARTESIAN_POINT('Ctrl Pts',(-13.2405097422111,5.89538421520699,0.598528395292872));
#3561=CARTESIAN_POINT('Ctrl Pts',(-13.3843290142384,5.91644376021923,0.374461997536319));
#3562=CARTESIAN_POINT('Ctrl Pts',(-13.4296642190767,5.92460700580665,0.119574227573619));
#3563=CARTESIAN_POINT('Ctrl Pts',(-13.4296253182383,5.92459115482435,-0.119766755586355));
#3564=CARTESIAN_POINT('Ctrl Pts',(-13.3842922335101,5.91641359576347,-0.374669709501813));
#3565=CARTESIAN_POINT('Ctrl Pts',(-13.2403979589254,5.8953456496019,-0.59872322823422));
#3566=CARTESIAN_POINT('Ctrl Pts',(-13.0676299873348,5.87508873599765,-0.780322400839761));
#3567=CARTESIAN_POINT('Ctrl Pts',(-12.9554220717229,5.86407660437688,-0.861625103513371));
#3568=CARTESIAN_POINT('Ctrl Pts',(-12.7024805472264,5.84815795494093,-0.971855454462235));
#3569=CARTESIAN_POINT('Ctrl Pts',(-12.5625041534178,5.84382474976352,-0.999141215193046));
#3570=CARTESIAN_POINT('Ctrl Pts',(-12.1981657362553,5.8432976608614,-1.00166254046375));
#3571=CARTESIAN_POINT('Ctrl Pts',(-11.9112711559271,5.86144665456792,-0.892429708902027));
#3572=CARTESIAN_POINT('Ctrl Pts',(-11.7282408997332,5.88272399126246,-0.712069056663859));
#3573=CARTESIAN_POINT('Ctrl Pts',(-11.6199843395186,5.89533514353784,-0.599014799133686));
#3574=CARTESIAN_POINT('Ctrl Pts',(-11.5121688868997,5.91109120383654,-0.430441231608476));
#3575=CARTESIAN_POINT('Ctrl Pts',(-11.4506970319975,5.92117313680743,-0.214808848136133));
#3576=CARTESIAN_POINT('Ctrl Pts',(-11.4336896339877,5.92399750826545,-0.0903772556247663));
#3577=CARTESIAN_POINT('Ctrl Pts',(-11.4253395813362,5.92549348750944,0.0887516303553966));
#3578=CARTESIAN_POINT('Ctrl Pts',(-11.4759391586775,5.91645238097389,0.373789699542128));
#3579=CARTESIAN_POINT('Ctrl Pts',(-11.6202170398282,5.8952920634098,0.598790738714452));
#3580=CARTESIAN_POINT('Ctrl Pts',(-11.792884701926,5.87507217891444,0.780167119997466));
#3581=CARTESIAN_POINT('Ctrl Pts',(-11.9051374289599,5.86405115731345,0.861525029957537));
#3582=CARTESIAN_POINT('Ctrl Pts',(-12.1579479395019,5.84817833435726,0.971521909353962));
#3583=CARTESIAN_POINT('Ctrl Pts',(-12.2983549564728,5.84371839234553,0.999392548488257));
#3584=CARTESIAN_POINT('Ctrl Pts',(-12.4302293937643,5.84371822200836,0.999392733607483));
#3585=CARTESIAN_POINT('',(-12.4302293937643,5.84422216200635,1.));
#3586=CARTESIAN_POINT('',(-12.4302293937643,6.08890895085005,1.29485665783831));
#3587=CARTESIAN_POINT('',(-13.4302293891297,5.92521705509939,-9.62763526687191E-5));
#3588=CARTESIAN_POINT('Ctrl Pts',(-12.4302293937643,5.84422216200635,0.999999999999999));
#3589=CARTESIAN_POINT('Ctrl Pts',(-12.4592320214116,5.84422216200635,0.999999999999999));
#3590=CARTESIAN_POINT('Ctrl Pts',(-12.4886478834784,5.8444442230921,0.998734139041022));
#3591=CARTESIAN_POINT('Ctrl Pts',(-12.5182411890796,5.84487442357384,0.996119432540782));
#3592=CARTESIAN_POINT('Ctrl Pts',(-12.5476087369448,5.84530134219555,0.993524672788903));
#3593=CARTESIAN_POINT('Ctrl Pts',(-12.5771503766343,5.84593323667031,0.989601419867018));
#3594=CARTESIAN_POINT('Ctrl Pts',(-12.6066265082011,5.84675650149613,0.984319083437057));
#3595=CARTESIAN_POINT('Ctrl Pts',(-12.6360181252477,5.84757740584151,0.979051892621711));
#3596=CARTESIAN_POINT('Ctrl Pts',(-12.6653439314479,5.84858858470984,0.972433382071454));
#3597=CARTESIAN_POINT('Ctrl Pts',(-12.6943672114053,5.84977654929374,0.96448494715668));
#3598=CARTESIAN_POINT('Ctrl Pts',(-12.7233731679207,5.85096380480425,0.956541256511066));
#3599=CARTESIAN_POINT('Ctrl Pts',(-12.7520762879357,5.85232763505328,0.94726936028975));
#3600=CARTESIAN_POINT('Ctrl Pts',(-12.7802512593826,5.85385457537269,0.936741529766411));
#3601=CARTESIAN_POINT('Ctrl Pts',(-12.7967306907133,5.85474767683288,0.930583842597197));
#3602=CARTESIAN_POINT('Ctrl Pts',(-12.8130297003045,5.85569657881332,0.923997448220513));
#3603=CARTESIAN_POINT('Ctrl Pts',(-12.8291063084377,5.8566985871014,0.917004474874906));
#3604=CARTESIAN_POINT('Ctrl Pts',(-12.8575304396385,5.85847018063709,0.904640598725699));
#3605=CARTESIAN_POINT('Ctrl Pts',(-12.8853056660692,5.86040778318034,0.890982659342418));
#3606=CARTESIAN_POINT('Ctrl Pts',(-12.9122329134691,5.86246204056025,0.876169279872447));
#3607=CARTESIAN_POINT('Ctrl Pts',(-12.939327595744,5.86452907140796,0.861263790120844));
#3608=CARTESIAN_POINT('Ctrl Pts',(-12.9655631808851,5.86671421233306,0.845188887893915));
#3609=CARTESIAN_POINT('Ctrl Pts',(-12.9907703544572,5.86896718276849,0.828126700080028));
#3610=CARTESIAN_POINT('Ctrl Pts',(-13.0161011819465,5.87123120516175,0.810980813617723));
#3611=CARTESIAN_POINT('Ctrl Pts',(-13.040393080685,5.87356372417359,0.792838498440963));
#3612=CARTESIAN_POINT('Ctrl Pts',(-13.0635150989357,5.87591371564642,0.773918093615534));
#3613=CARTESIAN_POINT('Ctrl Pts',(-13.0869035542154,5.87829078627554,0.754779667318463));
#3614=CARTESIAN_POINT('Ctrl Pts',(-13.1090947171264,5.88068573435905,0.734845746588785));
#3615=CARTESIAN_POINT('Ctrl Pts',(-13.1300001719029,5.88304575146868,0.714367453110294));
#3616=CARTESIAN_POINT('Ctrl Pts',(-13.1383433794932,5.88398761630122,0.706194722336734));
#3617=CARTESIAN_POINT('Ctrl Pts',(-13.1464823508734,5.88492391751257,0.6979355119476));
#3618=CARTESIAN_POINT('Ctrl Pts',(-13.1544136476108,5.88585129831765,0.689606530190082));
#3619=CARTESIAN_POINT('Ctrl Pts',(-13.1760213569284,5.88837781769102,0.666915383623946));
#3620=CARTESIAN_POINT('Ctrl Pts',(-13.1967993780494,5.89093180677019,0.642953073760821));
#3621=CARTESIAN_POINT('Ctrl Pts',(-13.2165148917462,5.893455949781,0.617863347078739));
#3622=CARTESIAN_POINT('Ctrl Pts',(-13.235525524171,5.89588984806556,0.59367064386409));
#3623=CARTESIAN_POINT('Ctrl Pts',(-13.2535478793342,5.89829599628131,0.568430356987537));
#3624=CARTESIAN_POINT('Ctrl Pts',(-13.270406707377,5.90062300904914,0.54231179379622));
#3625=CARTESIAN_POINT('Ctrl Pts',(-13.2872366276282,5.90294603169379,0.516238016042039));
#3626=CARTESIAN_POINT('Ctrl Pts',(-13.302906563573,5.90519019004457,0.489289499082407));
#3627=CARTESIAN_POINT('Ctrl Pts',(-13.3172825639117,5.9073043626005,0.461667275569134));
#3628=CARTESIAN_POINT('Ctrl Pts',(-13.331660445953,5.90941881188457,0.434041436529585));
#3629=CARTESIAN_POINT('Ctrl Pts',(-13.3447437328419,5.9114032413434,0.405742328697114));
#3630=CARTESIAN_POINT('Ctrl Pts',(-13.3564446413391,5.91320650939921,0.376995112912612));
#3631=CARTESIAN_POINT('Ctrl Pts',(-13.3577869138172,5.91341337171956,0.373697369273322));
#3632=CARTESIAN_POINT('Ctrl Pts',(-13.3591110475612,5.91361785003098,0.370393748670391));
#3633=CARTESIAN_POINT('Ctrl Pts',(-13.3604169514719,5.91381986712987,0.367084605351364));
#3634=CARTESIAN_POINT('Ctrl Pts',(-13.3723151401828,5.9156604601059,0.336934751784082));
#3635=CARTESIAN_POINT('Ctrl Pts',(-13.3827086173401,5.91729674366869,0.306293119193863));
#3636=CARTESIAN_POINT('Ctrl Pts',(-13.3915566759856,5.91871491003209,0.2754085264783));
#3637=CARTESIAN_POINT('Ctrl Pts',(-13.4004276260277,5.9201367454273,0.244444030194534));
#3638=CARTESIAN_POINT('Ctrl Pts',(-13.4077451239213,5.92133933355236,0.213236017734468));
#3639=CARTESIAN_POINT('Ctrl Pts',(-13.413520678218,5.92230875917455,0.182039143915082));
#3640=CARTESIAN_POINT('Ctrl Pts',(-13.4193449731899,5.92328636590921,0.15057899550552));
#3641=CARTESIAN_POINT('Ctrl Pts',(-13.4236012816078,5.92402685815631,0.119130873576328));
#3642=CARTESIAN_POINT('Ctrl Pts',(-13.4263543498779,5.92451596540413,0.0879492570048032));
#3643=CARTESIAN_POINT('Ctrl Pts',(-13.4289729319664,5.9249811799767,0.0582908487725101));
#3644=CARTESIAN_POINT('Ctrl Pts',(-13.4302321782768,5.9252189697697,0.028873943407611));
#3645=CARTESIAN_POINT('Ctrl Pts',(-13.4302293891297,5.92521705509939,-9.62763526685966E-5));
#3646=CARTESIAN_POINT('Ctrl Pts',(-13.4302293891297,5.92521705509939,-9.62763526688415E-5));
#3647=CARTESIAN_POINT('Ctrl Pts',(-13.4302264582134,5.92521504310856,-0.0305390195007855));
#3648=CARTESIAN_POINT('Ctrl Pts',(-13.4288294590287,5.92494889813534,-0.0614755629460699));
#3649=CARTESIAN_POINT('Ctrl Pts',(-13.4259265463018,5.9244327519576,-0.0926670406820359));
#3650=CARTESIAN_POINT('Ctrl Pts',(-13.4230403352885,5.92391957539228,-0.123679060342671));
#3651=CARTESIAN_POINT('Ctrl Pts',(-13.4186652254003,5.92315926607723,-0.154942467869905));
#3652=CARTESIAN_POINT('Ctrl Pts',(-13.4127399837538,5.92216571327227,-0.186206714590468));
#3653=CARTESIAN_POINT('Ctrl Pts',(-13.4068458877949,5.92117738301978,-0.21730662261883));
#3654=CARTESIAN_POINT('Ctrl Pts',(-13.3994178054916,5.91995825489446,-0.248406687039036));
#3655=CARTESIAN_POINT('Ctrl Pts',(-13.3904465693376,5.91852200028117,-0.279254320886848));
#3656=CARTESIAN_POINT('Ctrl Pts',(-13.3818241197141,5.9171415848248,-0.308902650759479));
#3657=CARTESIAN_POINT('Ctrl Pts',(-13.371776487637,5.915560597712,-0.338317213207077));
#3658=CARTESIAN_POINT('Ctrl Pts',(-13.3603408425699,5.91379117695691,-0.367277405785775));
#3659=CARTESIAN_POINT('Ctrl Pts',(-13.3485095199021,5.91196053358123,-0.397239631870212));
#3660=CARTESIAN_POINT('Ctrl Pts',(-13.3351782714556,5.90992819122401,-0.426748421701383));
#3661=CARTESIAN_POINT('Ctrl Pts',(-13.3204401056177,5.90775093729684,-0.455548996817583));
#3662=CARTESIAN_POINT('Ctrl Pts',(-13.3062511503052,5.90565481766999,-0.483276332619849));
#3663=CARTESIAN_POINT('Ctrl Pts',(-13.2907588121517,5.9034243853599,-0.510346745426924));
#3664=CARTESIAN_POINT('Ctrl Pts',(-13.2740937370534,5.90111031294684,-0.536556586135456));
#3665=CARTESIAN_POINT('Ctrl Pts',(-13.2574071915474,5.8987932592044,-0.562800194226458));
#3666=CARTESIAN_POINT('Ctrl Pts',(-13.2395453245768,5.89639234970513,-0.588180474034698));
#3667=CARTESIAN_POINT('Ctrl Pts',(-13.2206804853333,5.89395845313342,-0.612525160166824));
#3668=CARTESIAN_POINT('Ctrl Pts',(-13.2017317678401,5.89151373478996,-0.636978089450959));
#3669=CARTESIAN_POINT('Ctrl Pts',(-13.1817716774107,5.88903573538278,-0.660385759745594));
#3670=CARTESIAN_POINT('Ctrl Pts',(-13.1610090523917,5.88657600514603,-0.682613426864979));
#3671=CARTESIAN_POINT('Ctrl Pts',(-13.1587569437218,5.88630919977885,-0.685024447715524));
#3672=CARTESIAN_POINT('Ctrl Pts',(-13.156495420895,5.88604260935945,-0.687421627037074));
#3673=CARTESIAN_POINT('Ctrl Pts',(-13.1542247700728,5.88577629967664,-0.689804823905987));
#3674=CARTESIAN_POINT('Ctrl Pts',(-13.1339907182747,5.88340318098149,-0.711041787519624));
#3675=CARTESIAN_POINT('Ctrl Pts',(-13.1124165710007,5.88098167042095,-0.731808711400977));
#3676=CARTESIAN_POINT('Ctrl Pts',(-13.089570727107,5.87856224500728,-0.751843737851061));
#3677=CARTESIAN_POINT('Ctrl Pts',(-13.0670118937186,5.8761732146411,-0.771627065870116));
#3678=CARTESIAN_POINT('Ctrl Pts',(-13.043213336531,5.87378621735982,-0.790696138338821));
#3679=CARTESIAN_POINT('Ctrl Pts',(-13.018287850596,5.87144985155954,-0.808818429159916));
#3680=CARTESIAN_POINT('Ctrl Pts',(-12.9935019925622,5.86912657364263,-0.826839202303933));
#3681=CARTESIAN_POINT('Ctrl Pts',(-12.9676021277528,5.86685336153941,-0.843923179825897));
#3682=CARTESIAN_POINT('Ctrl Pts',(-12.9407418268909,5.86467800149521,-0.859870371406732));
#3683=CARTESIAN_POINT('Ctrl Pts',(-12.9140104238785,5.86251308062044,-0.875741035226008));
#3684=CARTESIAN_POINT('Ctrl Pts',(-12.8863282483644,5.86044507490852,-0.890485297091702));
#3685=CARTESIAN_POINT('Ctrl Pts',(-12.8578830598608,5.85852108594758,-0.903942665147648));
#3686=CARTESIAN_POINT('Ctrl Pts',(-12.8483500352163,5.85787628676904,-0.908452722140648));
#3687=CARTESIAN_POINT('Ctrl Pts',(-12.8387315828453,5.85724766305677,-0.91281857737988));
#3688=CARTESIAN_POINT('Ctrl Pts',(-12.8290355364334,5.85663698778019,-0.917035255903188));
#3689=CARTESIAN_POINT('Ctrl Pts',(-12.8006813737891,5.85485118917947,-0.929366095050314));
#3690=CARTESIAN_POINT('Ctrl Pts',(-12.7716621236898,5.85324772267947,-0.940417687690155));
#3691=CARTESIAN_POINT('Ctrl Pts',(-12.7421979764678,5.85183237825636,-0.950092418349892));
#3692=CARTESIAN_POINT('Ctrl Pts',(-12.7126954949783,5.85041519240232,-0.959779736297889));
#3693=CARTESIAN_POINT('Ctrl Pts',(-12.6827476165911,5.84918661845529,-0.968086386359692));
#3694=CARTESIAN_POINT('Ctrl Pts',(-12.6525913531979,5.84815246901999,-0.97496418344309));
#3695=CARTESIAN_POINT('Ctrl Pts',(-12.6223845035406,5.84711658482876,-0.981853517833188));
#3696=CARTESIAN_POINT('Ctrl Pts',(-12.5919692612567,5.84627577797941,-0.987309141862486));
#3697=CARTESIAN_POINT('Ctrl Pts',(-12.5615896425454,5.84563589037716,-0.991334698797625));
#3698=CARTESIAN_POINT('Ctrl Pts',(-12.5310315251629,5.84499224304745,-0.995383908319399));
#3699=CARTESIAN_POINT('Ctrl Pts',(-12.5005101422583,5.84455188294582,-0.997986271070962));
#3700=CARTESIAN_POINT('Ctrl Pts',(-12.4702692367735,5.84432075555793,-0.999198083951227));
#3701=CARTESIAN_POINT('Ctrl Pts',(-12.4567895079721,5.84421773170804,-0.999738243338723));
#3702=CARTESIAN_POINT('Ctrl Pts',(-12.4433653826999,5.84415627999187,-1.00000280430924));
#3703=CARTESIAN_POINT('Ctrl Pts',(-12.4300176179556,5.84413692696769,-0.999999977575504));
#3704=CARTESIAN_POINT('Ctrl Pts',(-12.3997273096931,5.84409300882263,-0.999993562820831));
#3705=CARTESIAN_POINT('Ctrl Pts',(-12.3690627220166,5.84432630738648,-0.998606698701212));
#3706=CARTESIAN_POINT('Ctrl Pts',(-12.3382632274432,5.84480595565223,-0.995762132365058));
#3707=CARTESIAN_POINT('Ctrl Pts',(-12.3075934980838,5.8452835830517,-0.992929550828145));
#3708=CARTESIAN_POINT('Ctrl Pts',(-12.2767906587517,5.84600548867243,-0.988651368556739));
#3709=CARTESIAN_POINT('Ctrl Pts',(-12.2460999634423,5.84694119401489,-0.9829020057408));
#3710=CARTESIAN_POINT('Ctrl Pts',(-12.2154843590106,5.8478746099685,-0.97716670988216));
#3711=CARTESIAN_POINT('Ctrl Pts',(-12.1849810389625,5.8490207807168,-0.969967418608316));
#3712=CARTESIAN_POINT('Ctrl Pts',(-12.1548321948058,5.85034945092846,-0.961330527345209));
#3713=CARTESIAN_POINT('Ctrl Pts',(-12.1247087433682,5.85167700207402,-0.952700910462241));
#3714=CARTESIAN_POINT('Ctrl Pts',(-12.094939848471,5.85318674539381,-0.942636261039028));
#3715=CARTESIAN_POINT('Ctrl Pts',(-12.0657555508963,5.85484850193932,-0.931213626331269));
#3716=CARTESIAN_POINT('Ctrl Pts',(-12.0364962427691,5.85651452959249,-0.91976163274865));
#3717=CARTESIAN_POINT('Ctrl Pts',(-12.0078251817651,5.85833335289554,-0.906944943031127));
#3718=CARTESIAN_POINT('Ctrl Pts',(-11.9799526239205,5.86027455960027,-0.892889035960829));
#3719=CARTESIAN_POINT('Ctrl Pts',(-11.9520165849043,5.86222018750224,-0.878801115845509));
#3720=CARTESIAN_POINT('Ctrl Pts',(-11.9248832439706,5.86428875690958,-0.863468752525495));
#3721=CARTESIAN_POINT('Ctrl Pts',(-11.8987336381442,5.86644964730411,-0.847060955160747));
#3722=CARTESIAN_POINT('Ctrl Pts',(-11.8723903943151,5.8686265391062,-0.83053165794883));
#3723=CARTESIAN_POINT('Ctrl Pts',(-11.8470459767866,5.87089712423285,-0.812911460103129));
#3724=CARTESIAN_POINT('Ctrl Pts',(-11.8228465976897,5.87323009688088,-0.794409301954961));
#3725=CARTESIAN_POINT('Ctrl Pts',(-11.8066067163169,5.874795723788,-0.781992749767297));
#3726=CARTESIAN_POINT('Ctrl Pts',(-11.7908816808213,5.87638944737418,-0.769179747345653));
#3727=CARTESIAN_POINT('Ctrl Pts',(-11.7757046159195,5.87800180612318,-0.756040551284902));
#3728=CARTESIAN_POINT('Ctrl Pts',(-11.7563448014304,5.88005852568473,-0.739280235643044));
#3729=CARTESIAN_POINT('Ctrl Pts',(-11.7378440338808,5.88214556739628,-0.72195704287926));
#3730=CARTESIAN_POINT('Ctrl Pts',(-11.720315065076,5.88417207266275,-0.704288041871364));
#3731=CARTESIAN_POINT('Ctrl Pts',(-11.7155619706134,5.8847215728112,-0.699496976761671));
#3732=CARTESIAN_POINT('Ctrl Pts',(-11.7108800779854,5.88526662196504,-0.694680646620972));
#3733=CARTESIAN_POINT('Ctrl Pts',(-11.7062710700307,5.88580540867468,-0.689843710920692));
#3734=CARTESIAN_POINT('Ctrl Pts',(-11.6846649679798,5.88833113237632,-0.667169129453078));
#3735=CARTESIAN_POINT('Ctrl Pts',(-11.6638747133822,5.89088291055031,-0.643210366431919));
#3736=CARTESIAN_POINT('Ctrl Pts',(-11.6441426510202,5.89340475457111,-0.618116196909614));
#3737=CARTESIAN_POINT('Ctrl Pts',(-11.6254120599292,5.8957986061758,-0.594295644375904));
#3738=CARTESIAN_POINT('Ctrl Pts',(-11.6076352765853,5.89816548504561,-0.569452789017778));
#3739=CARTESIAN_POINT('Ctrl Pts',(-11.590985695849,5.90045750206494,-0.543755474004179));
#3740=CARTESIAN_POINT('Ctrl Pts',(-11.5743648229732,5.90274556709859,-0.51810246730951));
#3741=CARTESIAN_POINT('Ctrl Pts',(-11.5588677091084,5.90495902821867,-0.491598471425702));
#3742=CARTESIAN_POINT('Ctrl Pts',(-11.5446263223345,5.90705024359962,-0.464442891940597));
#3743=CARTESIAN_POINT('Ctrl Pts',(-11.5303801053463,5.90914216825267,-0.437278102167764));
#3744=CARTESIAN_POINT('Ctrl Pts',(-11.5173907847708,5.91111176422898,-0.409461898920433));
#3745=CARTESIAN_POINT('Ctrl Pts',(-11.5057441424055,5.91291134121083,-0.381217811782318));
#3746=CARTESIAN_POINT('Ctrl Pts',(-11.5038371418876,5.91320600074693,-0.376593175160707));
#3747=CARTESIAN_POINT('Ctrl Pts',(-11.5019660327003,5.91349610203886,-0.371957106866477));
#3748=CARTESIAN_POINT('Ctrl Pts',(-11.5001310654575,5.91378143573301,-0.367310631047959));
#3749=CARTESIAN_POINT('Ctrl Pts',(-11.4853063383237,5.91608665081212,-0.32977168510081));
#3750=CARTESIAN_POINT('Ctrl Pts',(-11.4728396786202,5.91808068251128,-0.291540832281319));
#3751=CARTESIAN_POINT('Ctrl Pts',(-11.4627498179488,5.91971698624287,-0.252949145837491));
#3752=CARTESIAN_POINT('Ctrl Pts',(-11.4567469422105,5.92069049106031,-0.229989354240704));
#3753=CARTESIAN_POINT('Ctrl Pts',(-11.4515843367821,5.92153737618263,-0.206901800000682));
#3754=CARTESIAN_POINT('Ctrl Pts',(-11.4472572995214,5.92224784012799,-0.183754896369219));
#3755=CARTESIAN_POINT('Ctrl Pts',(-11.4432489878082,5.9229059719587,-0.162312972170666));
#3756=CARTESIAN_POINT('Ctrl Pts',(-11.439961640438,5.92344703975218,-0.140819734786591));
#3757=CARTESIAN_POINT('Ctrl Pts',(-11.4373971326886,5.92387645133334,-0.119516113420817));
#3758=CARTESIAN_POINT('Ctrl Pts',(-11.4362507877717,5.92406839997666,-0.109993311990914));
#3759=CARTESIAN_POINT('Ctrl Pts',(-11.435248171785,5.92423803831645,-0.100508449595123));
#3760=CARTESIAN_POINT('Ctrl Pts',(-11.4343860977113,5.92438584936314,-0.0910830923183082));
#3761=CARTESIAN_POINT('Ctrl Pts',(-11.4327073810137,5.92467368178929,-0.0727290956907958));
#3762=CARTESIAN_POINT('Ctrl Pts',(-11.4315567599486,5.92487874563008,-0.0546031136597995));
#3763=CARTESIAN_POINT('Ctrl Pts',(-11.4308953682944,5.92499615025902,-0.0364898004670366));
#3764=CARTESIAN_POINT('Ctrl Pts',(-11.4304572876631,5.92507391461186,-0.0244922319640955));
#3765=CARTESIAN_POINT('Ctrl Pts',(-11.4302349158949,5.92511322082742,-0.0125000346912251));
#3766=CARTESIAN_POINT('Ctrl Pts',(-11.4302294949532,5.92511264772102,-0.000449864268245586));
#3767=CARTESIAN_POINT('Ctrl Pts',(-11.4302143732044,5.92511104903731,0.0331641574895805));
#3768=CARTESIAN_POINT('Ctrl Pts',(-11.4318977520128,5.9247991356592,0.067213468042801));
#3769=CARTESIAN_POINT('Ctrl Pts',(-11.4353878553072,5.92419264473191,0.101441181777182));
#3770=CARTESIAN_POINT('Ctrl Pts',(-11.4388626723955,5.92358881015732,0.135518982502963));
#3771=CARTESIAN_POINT('Ctrl Pts',(-11.4441286896916,5.92269297280656,0.169773014320252));
#3772=CARTESIAN_POINT('Ctrl Pts',(-11.4512443561658,5.92152066394918,0.203932087122808));
#3773=CARTESIAN_POINT('Ctrl Pts',(-11.4583297414214,5.92035334393449,0.237945793591238));
#3774=CARTESIAN_POINT('Ctrl Pts',(-11.467249192492,5.91891190049415,0.271864682626153));
#3775=CARTESIAN_POINT('Ctrl Pts',(-11.4780094169704,5.91721166745705,0.305413024926134));
#3776=CARTESIAN_POINT('Ctrl Pts',(-11.4846501746176,5.91616235518983,0.326117649734809));
#3777=CARTESIAN_POINT('Ctrl Pts',(-11.4919910334845,5.91501447413545,0.346681019744403));
#3778=CARTESIAN_POINT('Ctrl Pts',(-11.5000236454424,5.91377162874814,0.367038507229061));
#3779=CARTESIAN_POINT('Ctrl Pts',(-11.5110521468223,5.91206524455569,0.394988641007747));
#3780=CARTESIAN_POINT('Ctrl Pts',(-11.5233988641988,5.91017984926752,0.422578110632233));
#3781=CARTESIAN_POINT('Ctrl Pts',(-11.5369898164793,5.90816323008511,0.449580979993369));
#3782=CARTESIAN_POINT('Ctrl Pts',(-11.5505815991783,5.90614648768562,0.476585499252034));
#3783=CARTESIAN_POINT('Ctrl Pts',(-11.5654174905502,5.90399850535563,0.503002719000625));
#3784=CARTESIAN_POINT('Ctrl Pts',(-11.5813761495079,5.90176707905666,0.528628574440787));
#3785=CARTESIAN_POINT('Ctrl Pts',(-11.5973542760978,5.89953293068769,0.554285690322862));
#3786=CARTESIAN_POINT('Ctrl Pts',(-11.6144574953387,5.8972151346425,0.579148962563932));
#3787=CARTESIAN_POINT('Ctrl Pts',(-11.6325217821314,5.89486166201193,0.603044414900698));
#3788=CARTESIAN_POINT('Ctrl Pts',(-11.6506773225831,5.89249630056497,0.627060577647201));
#3789=CARTESIAN_POINT('Ctrl Pts',(-11.6698031472941,5.89009490117412,0.650098664204443));
#3790=CARTESIAN_POINT('Ctrl Pts',(-11.689697113958,5.88770616560203,0.672020790277225));
#3791=CARTESIAN_POINT('Ctrl Pts',(-11.695162664264,5.88704989857104,0.678043545059696));
#3792=CARTESIAN_POINT('Ctrl Pts',(-11.700686012957,5.88639458738996,0.683982313641876));
#3793=CARTESIAN_POINT('Ctrl Pts',(-11.7062625862806,5.88574124196773,0.689834807516864));
#3794=CARTESIAN_POINT('Ctrl Pts',(-11.7263477798429,5.88338808197015,0.710913786574672));
#3795=CARTESIAN_POINT('Ctrl Pts',(-11.7477609028786,5.88098567143924,0.731537493965504));
#3796=CARTESIAN_POINT('Ctrl Pts',(-11.770433452944,5.87858424746972,0.751444819316098));
#3797=CARTESIAN_POINT('Ctrl Pts',(-11.7928148101204,5.87621366597628,0.771096466696523));
#3798=CARTESIAN_POINT('Ctrl Pts',(-11.8164232274,5.87384404586535,0.7900493849918));
#3799=CARTESIAN_POINT('Ctrl Pts',(-11.8411460208529,5.87152371333848,0.808072261471275));
#3800=CARTESIAN_POINT('Ctrl Pts',(-11.8657285654887,5.86921654372107,0.825992896789759));
#3801=CARTESIAN_POINT('Ctrl Pts',(-11.8914125449874,5.86695810407126,0.842993422903399));
#3802=CARTESIAN_POINT('Ctrl Pts',(-11.9180447110984,5.8647959028048,0.858875340688263));
#3803=CARTESIAN_POINT('Ctrl Pts',(-11.9445485982909,5.86264411619401,0.874680760180534));
#3804=CARTESIAN_POINT('Ctrl Pts',(-11.9719910902365,5.86058764309823,0.889377824348961));
#3805=CARTESIAN_POINT('Ctrl Pts',(-12.0001849714123,5.85867330873447,0.902807728591163));
#3806=CARTESIAN_POINT('Ctrl Pts',(-12.0104845902071,5.85797397563912,0.907713860289824));
#3807=CARTESIAN_POINT('Ctrl Pts',(-12.0208841714127,5.85729361156878,0.91245127650592));
#3808=CARTESIAN_POINT('Ctrl Pts',(-12.0313735835027,5.85663449938017,0.91701365454424));
#3809=CARTESIAN_POINT('Ctrl Pts',(-12.0589221689359,5.85490345780396,0.928995933444965));
#3810=CARTESIAN_POINT('Ctrl Pts',(-12.0871215827979,5.85333759236008,0.939780299010638));
#3811=CARTESIAN_POINT('Ctrl Pts',(-12.1157570467819,5.85194708130452,0.949266634293753));
#3812=CARTESIAN_POINT('Ctrl Pts',(-12.1444268796063,5.85055490133058,0.958764355260822));
#3813=CARTESIAN_POINT('Ctrl Pts',(-12.1735331620478,5.84933849692505,0.966960697313565));
#3814=CARTESIAN_POINT('Ctrl Pts',(-12.2028436425206,5.84830808303634,0.973804764894563));
#3815=CARTESIAN_POINT('Ctrl Pts',(-12.2322083633487,5.84727576232065,0.98066149772876));
#3816=CARTESIAN_POINT('Ctrl Pts',(-12.261777353607,5.84643012112625,0.986160875941255));
#3817=CARTESIAN_POINT('Ctrl Pts',(-12.2913103809521,5.84578143121621,0.990303745261672));
#3818=CARTESIAN_POINT('Ctrl Pts',(-12.3210469485782,5.84512827056483,0.994475167048973));
#3819=CARTESIAN_POINT('Ctrl Pts',(-12.3507463670084,5.8446747853114,0.997271376916708));
#3820=CARTESIAN_POINT('Ctrl Pts',(-12.3801670394779,5.84443146106362,0.998746094201777));
#3821=CARTESIAN_POINT('Ctrl Pts',(-12.3969595494538,5.84429257828103,0.999587822233208));
#3822=CARTESIAN_POINT('Ctrl Pts',(-12.4136613750755,5.84422216200635,0.999999999999999));
#3823=CARTESIAN_POINT('Ctrl Pts',(-12.4302293937643,5.84422216200635,0.999999999999999));
#3824=CARTESIAN_POINT('Origin',(-12.4302293937643,0.,0.));
#3825=CARTESIAN_POINT('',(-13.4302293937643,4.5,-6.73555739531044E-16));
#3826=CARTESIAN_POINT('Origin',(-12.4302293937643,4.5,-5.51091059616309E-16));
#3827=CARTESIAN_POINT('',(-13.4302293937643,1.49975978266185E-32,1.22464679914735E-16));
#3828=CARTESIAN_POINT('Ctrl Pts',(-12.4302293937643,1.29489435381091,-6.0889402328518));
#3829=CARTESIAN_POINT('Ctrl Pts',(-12.5942565650519,1.29489432255619,-6.08894022144968));
#3830=CARTESIAN_POINT('Ctrl Pts',(-12.9434847664517,1.22941870144897,-6.10373432775123));
#3831=CARTESIAN_POINT('Ctrl Pts',(-13.2352135646621,1.03138926022157,-6.14034164499865));
#3832=CARTESIAN_POINT('Ctrl Pts',(-13.4649707254284,0.802539126833306,-6.17429853801347));
#3833=CARTESIAN_POINT('Ctrl Pts',(-13.6645538759468,0.510108161031878,-6.21087860035388));
#3834=CARTESIAN_POINT('Ctrl Pts',(-13.7382347656975,0.121768500013446,-6.2270006516547));
#3835=CARTESIAN_POINT('Ctrl Pts',(-13.722307002809,-0.206473102178789,-6.22359662674633));
#3836=CARTESIAN_POINT('Ctrl Pts',(-13.639475073467,-0.54967950795853,-6.20621767344192));
#3837=CARTESIAN_POINT('Ctrl Pts',(-13.4650599641877,-0.802298136921999,
-6.17429031658926));
#3838=CARTESIAN_POINT('Ctrl Pts',(-13.2351717858284,-1.03178961021895,-6.14014988493062));
#3839=CARTESIAN_POINT('Ctrl Pts',(-13.0895235534449,-1.13087278981698,-6.12193678986932));
#3840=CARTESIAN_POINT('Ctrl Pts',(-12.8085826603911,-1.24610737129426,-6.09931038796544));
#3841=CARTESIAN_POINT('Ctrl Pts',(-12.5543859913687,-1.30578995791277,-6.08658018368838));
#3842=CARTESIAN_POINT('Ctrl Pts',(-12.0552211457951,-1.28477538936707,-6.09114347875703));
#3843=CARTESIAN_POINT('Ctrl Pts',(-11.6810858915091,-1.09012014643369,-6.13128471453802));
#3844=CARTESIAN_POINT('Ctrl Pts',(-11.4246965219914,-0.830211081602218,
-6.16997769478043));
#3845=CARTESIAN_POINT('Ctrl Pts',(-11.2673613307636,-0.624855866522035,
-6.19690899075049));
#3846=CARTESIAN_POINT('Ctrl Pts',(-11.0920011380406,-0.125799266344306,
-6.23306766503593));
#3847=CARTESIAN_POINT('Ctrl Pts',(-11.1298693974023,0.254022871674497,-6.22462921167978));
#3848=CARTESIAN_POINT('Ctrl Pts',(-11.2951627568963,0.657046732135944,-6.19244771333686));
#3849=CARTESIAN_POINT('Ctrl Pts',(-11.3950769811324,0.801381093653546,-6.17436843941782));
#3850=CARTESIAN_POINT('Ctrl Pts',(-11.6251524041765,1.03086438702109,-6.14021337372633));
#3851=CARTESIAN_POINT('Ctrl Pts',(-11.7709112212583,1.13013251926196,-6.12202566624175));
#3852=CARTESIAN_POINT('Ctrl Pts',(-12.0914404061413,1.26217657193465,-6.09612077171828));
#3853=CARTESIAN_POINT('Ctrl Pts',(-12.2662022355639,1.29489435617836,-6.08894022430558));
#3854=CARTESIAN_POINT('Ctrl Pts',(-12.4302293937643,1.29489435381091,-6.0889402328518));
#3855=CARTESIAN_POINT('Ctrl Pts',(-12.4302293937643,1.19652398778682,-6.00730758749701));
#3856=CARTESIAN_POINT('Ctrl Pts',(-12.5835260128158,1.19660554925645,-6.00733734217367));
#3857=CARTESIAN_POINT('Ctrl Pts',(-12.9099794791603,1.1339456710644,-6.02027410479885));
#3858=CARTESIAN_POINT('Ctrl Pts',(-13.1793649483868,0.947760265143857,-6.05208309125148));
#3859=CARTESIAN_POINT('Ctrl Pts',(-13.390127239501,0.734644744099366,-6.08145723820567));
#3860=CARTESIAN_POINT('Ctrl Pts',(-13.5712908603111,0.464550273602845,-6.11289252680422));
#3861=CARTESIAN_POINT('Ctrl Pts',(-13.6372762454486,0.110863463753234,-6.12664471204441));
#3862=CARTESIAN_POINT('Ctrl Pts',(-13.6230233985846,-0.188078828642945,
-6.12375264534608));
#3863=CARTESIAN_POINT('Ctrl Pts',(-13.5485622985786,-0.501106347863059,
-6.10889585516032));
#3864=CARTESIAN_POINT('Ctrl Pts',(-13.3901851790633,-0.734519663395452,
-6.08143345776283));
#3865=CARTESIAN_POINT('Ctrl Pts',(-13.1793404196312,-0.948112795692235,
-6.05190225429682));
#3866=CARTESIAN_POINT('Ctrl Pts',(-13.0448314929934,-1.04131898524137,-6.03606502647125));
#3867=CARTESIAN_POINT('Ctrl Pts',(-12.7836826024607,-1.15012783687734,-6.0163867285));
#3868=CARTESIAN_POINT('Ctrl Pts',(-12.5464205975656,-1.20689836538162,-6.00524419490769));
#3869=CARTESIAN_POINT('Ctrl Pts',(-12.0794526073123,-1.18675056022211,-6.00927493048454));
#3870=CARTESIAN_POINT('Ctrl Pts',(-11.7321555677729,-1.00228782075479,-6.04426997438495));
#3871=CARTESIAN_POINT('Ctrl Pts',(-11.4971890642621,-0.760513752850325,
-6.07766139091982));
#3872=CARTESIAN_POINT('Ctrl Pts',(-11.3537752566932,-0.570286282304659,
-6.10091025389764));
#3873=CARTESIAN_POINT('Ctrl Pts',(-11.1959278067123,-0.113851829768248,
-6.1318171205129));
#3874=CARTESIAN_POINT('Ctrl Pts',(-11.2298363795958,0.230967119360158,-6.12460974003898));
#3875=CARTESIAN_POINT('Ctrl Pts',(-11.3791293387795,0.600065235007544,-6.09708188247935));
#3876=CARTESIAN_POINT('Ctrl Pts',(-11.4699934418307,0.733649918402728,-6.08148733752786));
#3877=CARTESIAN_POINT('Ctrl Pts',(-11.6809686581905,0.947165898685803,-6.0519761018612));
#3878=CARTESIAN_POINT('Ctrl Pts',(-11.8155823945189,1.04056140059047,-6.03616052651344));
#3879=CARTESIAN_POINT('Ctrl Pts',(-12.1135732968508,1.16533663101808,-6.01359382211873));
#3880=CARTESIAN_POINT('Ctrl Pts',(-12.2768986229754,1.19651780974642,-6.00732988949686));
#3881=CARTESIAN_POINT('Ctrl Pts',(-12.4302293937643,1.19652398778682,-6.00730758749701));
#3882=CARTESIAN_POINT('Ctrl Pts',(-12.4302293937643,1.09815362176272,-5.92567494214221));
#3883=CARTESIAN_POINT('Ctrl Pts',(-12.5728768111359,1.09807191176829,-5.92564513328179));
#3884=CARTESIAN_POINT('Ctrl Pts',(-12.8764400238043,1.03857307634312,-5.93677323915331));
#3885=CARTESIAN_POINT('Ctrl Pts',(-13.1236421530229,0.863834068887647,-5.9638111997203));
#3886=CARTESIAN_POINT('Ctrl Pts',(-13.3152938488915,0.666818346565923,-5.98856002821125));
#3887=CARTESIAN_POINT('Ctrl Pts',(-13.4781043169547,0.419015044302822,-6.01490064545119));
#3888=CARTESIAN_POINT('Ctrl Pts',(-13.5363318958501,0.0999234953363876,
-6.02625541555216));
#3889=CARTESIAN_POINT('Ctrl Pts',(-13.5236242325651,-0.169584645174253,
-6.02383257520469));
#3890=CARTESIAN_POINT('Ctrl Pts',(-13.45763379556,-0.452598972368938,-6.011534802412));
#3891=CARTESIAN_POINT('Ctrl Pts',(-13.3153133841291,-0.666694064607999,
-5.98855204897587));
#3892=CARTESIAN_POINT('Ctrl Pts',(-13.1235487664965,-0.864416414698098,
-5.96366385619052));
#3893=CARTESIAN_POINT('Ctrl Pts',(-13.0002703379808,-0.951649292171483,
-5.95024248073981));
#3894=CARTESIAN_POINT('Ctrl Pts',(-12.7587075542712,-1.05425776004711,-5.93340511818793));
#3895=CARTESIAN_POINT('Ctrl Pts',(-12.5386313682688,-1.10804595290956,-5.92389983389524));
#3896=CARTESIAN_POINT('Ctrl Pts',(-12.1032856759994,-1.08903105885641,-5.92731281534742));
#3897=CARTESIAN_POINT('Ctrl Pts',(-11.7831058258753,-0.914801975659288,
-5.95717971506951));
#3898=CARTESIAN_POINT('Ctrl Pts',(-11.5695163116143,-0.690787431055235,
-5.98544778843915));
#3899=CARTESIAN_POINT('Ctrl Pts',(-11.4400693088082,-0.515889562697353,
-6.00490223026015));
#3900=CARTESIAN_POINT('Ctrl Pts',(-11.2997931554053,-0.101999726766142,
-6.03060418648155));
#3901=CARTESIAN_POINT('Ctrl Pts',(-11.3296621227584,0.20759284922966,-6.02466259409955));
#3902=CARTESIAN_POINT('Ctrl Pts',(-11.4632375981302,0.543731219297565,-6.0016238831943));
#3903=CARTESIAN_POINT('Ctrl Pts',(-11.5448774670807,0.665911891095343,-5.98861915101148));
#3904=CARTESIAN_POINT('Ctrl Pts',(-11.7368656075404,0.863751696770123,-5.96368471390795));
#3905=CARTESIAN_POINT('Ctrl Pts',(-11.8602650367562,0.951079271006522,-5.95028481323786));
#3906=CARTESIAN_POINT('Ctrl Pts',(-12.1357219210113,1.06855012001856,-5.93104620471383));
#3907=CARTESIAN_POINT('Ctrl Pts',(-12.2876161903209,1.09815981105343,-5.92565259953004));
#3908=CARTESIAN_POINT('Ctrl Pts',(-12.4302293937643,1.09815362176272,-5.92567494214221));
#3909=CARTESIAN_POINT('Ctrl Pts',(-12.4302293937643,0.99978325573863,-5.84404229678742));
#3910=CARTESIAN_POINT('Ctrl Pts',(-12.5621461601267,0.99978343577442,-5.8440423624668));
#3911=CARTESIAN_POINT('Ctrl Pts',(-12.8429347779986,0.943099924012935,-5.85331306554794));
#3912=CARTESIAN_POINT('Ctrl Pts',(-13.0677933839801,0.780205434661611,-5.87555266216742));
#3913=CARTESIAN_POINT('Ctrl Pts',(-13.2404503507067,0.598923881286639,-5.89571879628772));
#3914=CARTESIAN_POINT('Ctrl Pts',(-13.3848412084689,0.373457129363051,-5.91691457895316));
#3915=CARTESIAN_POINT('Ctrl Pts',(-13.4353733583957,0.0890185014896255,
-5.92589951644267));
#3916=CARTESIAN_POINT('Ctrl Pts',(-13.424340768652,-0.15119049294569,-5.92398868618882));
#3917=CARTESIAN_POINT('Ctrl Pts',(-13.3667210397683,-0.404025732400016,
-5.91421303176758));
#3918=CARTESIAN_POINT('Ctrl Pts',(-13.2404385953741,-0.59891564829936,-5.89569521995717));
#3919=CARTESIAN_POINT('Ctrl Pts',(-13.067717352081,-0.78073962392833,-5.8754162143469));
#3920=CARTESIAN_POINT('Ctrl Pts',(-12.9555781185883,-0.862095628303779,
-5.8643706575833));
#3921=CARTESIAN_POINT('Ctrl Pts',(-12.7338075873915,-0.958278092730466,
-5.85048152908445));
#3922=CARTESIAN_POINT('Ctrl Pts',(-12.5306657605727,-1.00915431280731,-5.84256385527983));
#3923=CARTESIAN_POINT('Ctrl Pts',(-12.1275176212317,-0.991005858992733,
-5.84544438068066));
#3924=CARTESIAN_POINT('Ctrl Pts',(-11.8341756471326,-0.82696922929531,-5.87016506660928));
#3925=CARTESIAN_POINT('Ctrl Pts',(-11.6420090545806,-0.621090137505721,
-5.89313135988199));
#3926=CARTESIAN_POINT('Ctrl Pts',(-11.5264833802844,-0.461319768593579,
-5.90890350468299));
#3927=CARTESIAN_POINT('Ctrl Pts',(-11.4037198985297,-0.0900521744392636,
-5.92935359629313));
#3928=CARTESIAN_POINT('Ctrl Pts',(-11.4296292764396,0.184537483648944,-5.92464303464332));
#3929=CARTESIAN_POINT('Ctrl Pts',(-11.5472040079934,0.486748936019,-5.9062581642446));
#3930=CARTESIAN_POINT('Ctrl Pts',(-11.6197939671611,0.598180724164063,-5.89573803344012));
#3931=CARTESIAN_POINT('Ctrl Pts',(-11.7926817635769,0.780052863263822,-5.87544750774877));
#3932=CARTESIAN_POINT('Ctrl Pts',(-11.9049361960917,0.861508044287461,-5.86441968634761));
#3933=CARTESIAN_POINT('Ctrl Pts',(-12.1578547926178,0.971710114229192,-5.84851928020843));
#3934=CARTESIAN_POINT('Ctrl Pts',(-12.2983125520166,0.999783242101451,-5.84404234601604));
#3935=CARTESIAN_POINT('Ctrl Pts',(-12.4302293937643,0.99978325573863,-5.84404229678742));
#3936=CARTESIAN_POINT('',(-12.4302293937643,1.,-5.84422216200635));
#3937=CARTESIAN_POINT('',(-12.4302293937643,1.29485665783831,-6.08890895085005));
#3938=CARTESIAN_POINT('',(-13.4302291165819,-0.00074455678695871,-5.92515607096498));
#3939=CARTESIAN_POINT('Ctrl Pts',(-12.4302293937643,1.,-5.84422216200635));
#3940=CARTESIAN_POINT('Ctrl Pts',(-12.5068876215205,1.,-5.84422216200635));
#3941=CARTESIAN_POINT('Ctrl Pts',(-12.583514447768,0.991164337845293,-5.84618803600395));
#3942=CARTESIAN_POINT('Ctrl Pts',(-12.734482852694,0.955797513292997,-5.85160509572529));
#3943=CARTESIAN_POINT('Ctrl Pts',(-12.8081512123687,0.92914750024174,-5.85522477680349));
#3944=CARTESIAN_POINT('Ctrl Pts',(-12.9239247195674,0.871137085216352,-5.86352598326324));
#3945=CARTESIAN_POINT('Ctrl Pts',(-12.9678164063148,0.844756284210404,-5.86723138398402));
#3946=CARTESIAN_POINT('Ctrl Pts',(-13.0616660207753,0.778065357329548,-5.87582109133897));
#3947=CARTESIAN_POINT('Ctrl Pts',(-13.1101602808476,0.736060124110439,-5.88069567821875));
#3948=CARTESIAN_POINT('Ctrl Pts',(-13.2147331458838,0.626288084301812,-5.89292243393707));
#3949=CARTESIAN_POINT('Ctrl Pts',(-13.26672687916,0.554987202036906,-5.90053924283666));
#3950=CARTESIAN_POINT('Ctrl Pts',(-13.329015288876,0.440435511458002,-5.90951215353627));
#3951=CARTESIAN_POINT('Ctrl Pts',(-13.3468856793851,0.401923730048892,-5.91211175363263));
#3952=CARTESIAN_POINT('Ctrl Pts',(-13.3850158785098,0.303849355425613,-5.91790597801221));
#3953=CARTESIAN_POINT('Ctrl Pts',(-13.4022161136297,0.243296810883259,-5.92076752333631));
#3954=CARTESIAN_POINT('Ctrl Pts',(-13.4247157097056,0.12137679578229,-5.9244956146738));
#3955=CARTESIAN_POINT('Ctrl Pts',(-13.4302746508587,0.0604058320419782,
-5.92539504948499));
#3956=CARTESIAN_POINT('Ctrl Pts',(-13.4302291165292,-0.00074462755025776,
-5.92532717514869));
#3957=CARTESIAN_POINT('Ctrl Pts',(-13.4302291165819,-0.00074455678695871,
-5.92515607096498));
#3958=CARTESIAN_POINT('Ctrl Pts',(-13.4302145007545,-0.0203747898610464,
-5.92516162275695));
#3959=CARTESIAN_POINT('Ctrl Pts',(-13.4296263010912,-0.0398710445290823,
-5.92506363544977));
#3960=CARTESIAN_POINT('Ctrl Pts',(-13.4284619148531,-0.0594292338889376,
-5.9248625596374));
#3961=CARTESIAN_POINT('Ctrl Pts',(-13.427825762458,-0.0701146822394427,
-5.92475270359868));
#3962=CARTESIAN_POINT('Ctrl Pts',(-13.4270167202947,-0.0808186195238017,
-5.92461207678402));
#3963=CARTESIAN_POINT('Ctrl Pts',(-13.4260278070042,-0.0915724859817269,
-5.92444075267486));
#3964=CARTESIAN_POINT('Ctrl Pts',(-13.4234433178898,-0.119677326989046,
-5.92399300331256));
#3965=CARTESIAN_POINT('Ctrl Pts',(-13.4196244803128,-0.148112331845129,
-5.9233355854986));
#3966=CARTESIAN_POINT('Ctrl Pts',(-13.4145053388056,-0.176637663064945,
-5.92247964262467));
#3967=CARTESIAN_POINT('Ctrl Pts',(-13.4094168909871,-0.204991960208965,
-5.92162883186987));
#3968=CARTESIAN_POINT('Ctrl Pts',(-13.4030435605191,-0.233434848039028,
-5.92058186957752));
#3969=CARTESIAN_POINT('Ctrl Pts',(-13.3953716865626,-0.261725724093029,
-5.91934969989586));
#3970=CARTESIAN_POINT('Ctrl Pts',(-13.3877346584708,-0.289888102201762,
-5.91812312676315));
#3971=CARTESIAN_POINT('Ctrl Pts',(-13.3788108949432,-0.317899175506962,
-5.91671302485451));
#3972=CARTESIAN_POINT('Ctrl Pts',(-13.3686383796453,-0.345526518834328,
-5.91513018986864));
#3973=CARTESIAN_POINT('Ctrl Pts',(-13.3659090692588,-0.352939001675285,
-5.91470551142476));
#3974=CARTESIAN_POINT('Ctrl Pts',(-13.363090150361,-0.360323920078094,-5.91426839858579));
#3975=CARTESIAN_POINT('Ctrl Pts',(-13.3601829769247,-0.367676941304649,
-5.91381905986056));
#3976=CARTESIAN_POINT('Ctrl Pts',(-13.348323638179,-0.397672389268568,-5.91198605599245));
#3977=CARTESIAN_POINT('Ctrl Pts',(-13.3349765249106,-0.427174288976912,
-5.90994960131782));
#3978=CARTESIAN_POINT('Ctrl Pts',(-13.3202356031391,-0.455948404180037,
-5.90776747673239));
#3979=CARTESIAN_POINT('Ctrl Pts',(-13.3055877002079,-0.484540947642264,
-5.90559912188955));
#3980=CARTESIAN_POINT('Ctrl Pts',(-13.289563906132,-0.512414264265203,-5.90328692976136));
#3981=CARTESIAN_POINT('Ctrl Pts',(-13.2723027529233,-0.539363011148032,
-5.90088759429642));
#3982=CARTESIAN_POINT('Ctrl Pts',(-13.254877178999,-0.566568457695916,-5.898465404017));
#3983=CARTESIAN_POINT('Ctrl Pts',(-13.2361909738944,-0.592831045617222,
-5.89595440233023));
#3984=CARTESIAN_POINT('Ctrl Pts',(-13.2164282067282,-0.617973645468872,
-5.89341291877673));
#3985=CARTESIAN_POINT('Ctrl Pts',(-13.1966654395621,-0.643116245320522,
-5.89087143522323));
#3986=CARTESIAN_POINT('Ctrl Pts',(-13.1758267003413,-0.667138450433701,
-5.888299469803));
#3987=CARTESIAN_POINT('Ctrl Pts',(-13.1541297156023,-0.689904576041336,
-5.88575535205665));
#3988=CARTESIAN_POINT('Ctrl Pts',(-13.1337114574319,-0.711328964535441,
-5.8833611736219));
#3989=CARTESIAN_POINT('Ctrl Pts',(-13.1119354995351,-0.732268036614787,
-5.88091652810431));
#3990=CARTESIAN_POINT('Ctrl Pts',(-13.0888693452294,-0.752458247568669,
-5.87847421176537));
#3991=CARTESIAN_POINT('Ctrl Pts',(-13.0660882115552,-0.772398974945793,
-5.87606207429961));
#3992=CARTESIAN_POINT('Ctrl Pts',(-13.0420487837158,-0.791608598781269,
-5.87365220880638));
#3993=CARTESIAN_POINT('Ctrl Pts',(-13.0168632956008,-0.809852249003558,
-5.87129547847511));
#3994=CARTESIAN_POINT('Ctrl Pts',(-12.9918183626218,-0.827994085088781,
-5.8689519005811));
#3995=CARTESIAN_POINT('Ctrl Pts',(-12.9656404510038,-0.845180103433922,
-5.86666086643067));
#3996=CARTESIAN_POINT('Ctrl Pts',(-12.9384829388873,-0.861207485957893,
-5.86447239238519));
#3997=CARTESIAN_POINT('Ctrl Pts',(-12.9114573425185,-0.877157016573312,
-5.86229454870192));
#3998=CARTESIAN_POINT('Ctrl Pts',(-12.8834621017052,-0.891958633552042,
-5.86021827118614));
#3999=CARTESIAN_POINT('Ctrl Pts',(-12.8546851894651,-0.905448660883642,
-5.85829285088076));
#4000=CARTESIAN_POINT('Ctrl Pts',(-12.8461436459829,-0.909452761603969,
-5.85772134893771));
#4001=CARTESIAN_POINT('Ctrl Pts',(-12.8375334567298,-0.913341579410674,
-5.85716313777255));
#4002=CARTESIAN_POINT('Ctrl Pts',(-12.8288600642316,-0.917111546412302,
-5.85661950636029));
#4003=CARTESIAN_POINT('Ctrl Pts',(-12.7961359807478,-0.931335359633967,
-5.85456842430408));
#4004=CARTESIAN_POINT('Ctrl Pts',(-12.7626532281845,-0.943801826616426,
-5.85275395442562));
#4005=CARTESIAN_POINT('Ctrl Pts',(-12.7286738356243,-0.954427008797875,
-5.85119022535545));
#4006=CARTESIAN_POINT('Ctrl Pts',(-12.6946247640078,-0.965073979263702,
-5.84962328966039));
#4007=CARTESIAN_POINT('Ctrl Pts',(-12.6600776972981,-0.973871960195361,
-5.84830812417968));
#4008=CARTESIAN_POINT('Ctrl Pts',(-12.6253069014017,-0.980787829254606,
-5.84725894463988));
#4009=CARTESIAN_POINT('Ctrl Pts',(-12.5940277649148,-0.98700921149949,-5.84631512298786));
#4010=CARTESIAN_POINT('Ctrl Pts',(-12.5625680645456,-0.991708188398394,
-5.84558654923866));
#4011=CARTESIAN_POINT('Ctrl Pts',(-12.531127836805,-0.994896730415759,-5.84508357217886));
#4012=CARTESIAN_POINT('Ctrl Pts',(-12.4973809048887,-0.998319209135062,
-5.84454369273739));
#4013=CARTESIAN_POINT('Ctrl Pts',(-12.4636986156402,-1.00000481725209,-5.8442637274595));
#4014=CARTESIAN_POINT('Ctrl Pts',(-12.4300857711154,-0.999999989686268,
-5.8442498696352));
#4015=CARTESIAN_POINT('Ctrl Pts',(-12.3964457198719,-0.999995158212949,
-5.84423600059418));
#4016=CARTESIAN_POINT('Ctrl Pts',(-12.3628741784227,-0.998297160738039,
-5.84448866996346));
#4017=CARTESIAN_POINT('Ctrl Pts',(-12.3293717699161,-0.994900869288844,
-5.84501408608402));
#4018=CARTESIAN_POINT('Ctrl Pts',(-12.2958961260104,-0.991507291088906,
-5.84553908245706));
#4019=CARTESIAN_POINT('Ctrl Pts',(-12.2624884600473,-0.98641801752302,-5.8463363899684));
#4020=CARTESIAN_POINT('Ctrl Pts',(-12.2291608584518,-0.979577176187413,
-5.84741220209162));
#4021=CARTESIAN_POINT('Ctrl Pts',(-12.2003045415045,-0.973654113131077,
-5.84834368152961));
#4022=CARTESIAN_POINT('Ctrl Pts',(-12.1714822894461,-0.966404873720001,
-5.84948394922433));
#4023=CARTESIAN_POINT('Ctrl Pts',(-12.1429321226033,-0.957841468085098,
-5.85079937270242));
#4024=CARTESIAN_POINT('Ctrl Pts',(-12.1144345913459,-0.949293850094169,
-5.85211237104285));
#4025=CARTESIAN_POINT('Ctrl Pts',(-12.0862088137393,-0.939437011609988,
-5.85359987992147));
#4026=CARTESIAN_POINT('Ctrl Pts',(-12.0584819453244,-0.928333902525599,
-5.85522845253844));
#4027=CARTESIAN_POINT('Ctrl Pts',(-12.0307493255855,-0.917228490347451,
-5.85685736296667));
#4028=CARTESIAN_POINT('Ctrl Pts',(-12.0035164563319,-0.904876542764548,
-5.8586273956604));
#4029=CARTESIAN_POINT('Ctrl Pts',(-11.976991236791,-0.891389462055422,-5.86050508300206));
#4030=CARTESIAN_POINT('Ctrl Pts',(-11.9503194013934,-0.877827832674227,
-5.86239314909809));
#4031=CARTESIAN_POINT('Ctrl Pts',(-11.9243636448556,-0.863118854449607,
-5.86439006323465));
#4032=CARTESIAN_POINT('Ctrl Pts',(-11.8993064649707,-0.847420110500802,
-5.86646179975291));
#4033=CARTESIAN_POINT('Ctrl Pts',(-11.8741364085495,-0.831650647506662,
-5.86854286894321));
#4034=CARTESIAN_POINT('Ctrl Pts',(-11.8498735094175,-0.814882991634751,
-5.87069943614703));
#4035=CARTESIAN_POINT('Ctrl Pts',(-11.8266657236187,-0.797314803625511,
-5.87289701379889));
#4036=CARTESIAN_POINT('Ctrl Pts',(-11.8031493349558,-0.779513004655496,
-5.875123813487));
#4037=CARTESIAN_POINT('Ctrl Pts',(-11.7807166929995,-0.760889825243683,
-5.87739272153807));
#4038=CARTESIAN_POINT('Ctrl Pts',(-11.759477199834,-0.74168153161429,-5.8796678562279));
#4039=CARTESIAN_POINT('Ctrl Pts',(-11.7407509176273,-0.724746102674908,
-5.88167378047139));
#4040=CARTESIAN_POINT('Ctrl Pts',(-11.7229515053941,-0.707356589426639,
-5.88368454497276));
#4041=CARTESIAN_POINT('Ctrl Pts',(-11.7061231638194,-0.689688457026103,
-5.88567555763584));
#4042=CARTESIAN_POINT('Ctrl Pts',(-11.6866581296135,-0.669252052166742,
-5.88797852548441));
#4043=CARTESIAN_POINT('Ctrl Pts',(-11.667818004418,-0.647733283425998,-5.89030237056838));
#4044=CARTESIAN_POINT('Ctrl Pts',(-11.649809623362,-0.625255933170801,-5.89260310173008));
#4045=CARTESIAN_POINT('Ctrl Pts',(-11.6318783158107,-0.602874783021202,
-5.89489398606472));
#4046=CARTESIAN_POINT('Ctrl Pts',(-11.6147721838589,-0.579543634374203,
-5.89716195390281));
#4047=CARTESIAN_POINT('Ctrl Pts',(-11.5986621529662,-0.555424093852063,
-5.89936357650184));
#4048=CARTESIAN_POINT('Ctrl Pts',(-11.58258732708,-0.53135726139663,-5.90156038792834));
#4049=CARTESIAN_POINT('Ctrl Pts',(-11.5675046859438,-0.506505991676054,
-5.90369114376546));
#4050=CARTESIAN_POINT('Ctrl Pts',(-11.5535435587647,-0.481063349997679,
-5.90571269936149));
#4051=CARTESIAN_POINT('Ctrl Pts',(-11.5488146310658,-0.472445391617939,
-5.90639744280163));
#4052=CARTESIAN_POINT('Ctrl Pts',(-11.5442140057291,-0.463759824048832,
-5.90706965748497));
#4053=CARTESIAN_POINT('Ctrl Pts',(-11.5397455322372,-0.45501482652746,-5.90772766671857));
#4054=CARTESIAN_POINT('Ctrl Pts',(-11.5249613802793,-0.426081596317538,
-5.9099047208103));
#4055=CARTESIAN_POINT('Ctrl Pts',(-11.5116020195662,-0.396446991709848,
-5.9119262752392));
#4056=CARTESIAN_POINT('Ctrl Pts',(-11.4997509995239,-0.366346772678213,
-5.91376075413862));
#4057=CARTESIAN_POINT('Ctrl Pts',(-11.4878540732106,-0.336129957032688,
-5.91560233910022));
#4058=CARTESIAN_POINT('Ctrl Pts',(-11.4774773723843,-0.305444596233139,
-5.91725539640872));
#4059=CARTESIAN_POINT('Ctrl Pts',(-11.4686542921061,-0.274542025691928,
-5.91868798183615));
#4060=CARTESIAN_POINT('Ctrl Pts',(-11.4600139155072,-0.244279369235048,
-5.92009090204234));
#4061=CARTESIAN_POINT('Ctrl Pts',(-11.4528632919579,-0.213809061728737,
-5.92128238665944));
#4062=CARTESIAN_POINT('Ctrl Pts',(-11.4471853155946,-0.183369409595853,
-5.92223243510267));
#4063=CARTESIAN_POINT('Ctrl Pts',(-11.4411101863144,-0.150800619216677,
-5.92324893583213));
#4064=CARTESIAN_POINT('Ctrl Pts',(-11.4367166701769,-0.118291409597998,
-5.92398904407821));
#4065=CARTESIAN_POINT('Ctrl Pts',(-11.4339211481789,-0.0858480039286165,
-5.92445833008817));
#4066=CARTESIAN_POINT('Ctrl Pts',(-11.431089721008,-0.0529879010954458,
-5.92493364352174));
#4067=CARTESIAN_POINT('Ctrl Pts',(-11.4298974125296,-0.0201943247625311,
-5.92513113326092));
#4068=CARTESIAN_POINT('Ctrl Pts',(-11.4303080569058,0.0125427307665045,
-5.92505658695115));
#4069=CARTESIAN_POINT('Ctrl Pts',(-11.4307185775025,0.0452699184545837,
-5.92498206311167));
#4070=CARTESIAN_POINT('Ctrl Pts',(-11.4327311014724,0.0779416178077606,
-5.92463566719669));
#4071=CARTESIAN_POINT('Ctrl Pts',(-11.4363609723752,0.110569258682268,-5.92402318161956));
#4072=CARTESIAN_POINT('Ctrl Pts',(-11.4399493805261,0.142824205370928,-5.92341769225201));
#4073=CARTESIAN_POINT('Ctrl Pts',(-11.4451185935596,0.175037037023386,-5.92255215740294));
#4074=CARTESIAN_POINT('Ctrl Pts',(-11.4519320204813,0.207205814174295,-5.92143216358902));
#4075=CARTESIAN_POINT('Ctrl Pts',(-11.4585455065396,0.23843059454462,-5.92034503613336));
#4076=CARTESIAN_POINT('Ctrl Pts',(-11.4667085178863,0.269614642654035,-5.91901816484915));
#4077=CARTESIAN_POINT('Ctrl Pts',(-11.4765205424234,0.300731486336286,-5.91745665873306));
#4078=CARTESIAN_POINT('Ctrl Pts',(-11.4834028145948,0.322557215218856,-5.91636139953884));
#4079=CARTESIAN_POINT('Ctrl Pts',(-11.491097239556,0.344349397393402,-5.91515070496908));
#4080=CARTESIAN_POINT('Ctrl Pts',(-11.4996492233318,0.366088167519528,-5.9138263380358));
#4081=CARTESIAN_POINT('Ctrl Pts',(-11.51159593145,0.396456179007265,-5.91197626142105));
#4082=CARTESIAN_POINT('Ctrl Pts',(-11.5250526304243,0.426287151505064,-5.90992593215957));
#4083=CARTESIAN_POINT('Ctrl Pts',(-11.539917668182,0.455351546929103,-5.90773166728562));
#4084=CARTESIAN_POINT('Ctrl Pts',(-11.5547892593215,0.484428755645817,-5.90553643505083));
#4085=CARTESIAN_POINT('Ctrl Pts',(-11.5710700779739,0.512738103043412,-5.90319714026504));
#4086=CARTESIAN_POINT('Ctrl Pts',(-11.5886129139444,0.540075643679213,-5.90077017447893));
#4087=CARTESIAN_POINT('Ctrl Pts',(-11.606228870658,0.567527130617118,-5.89833309279467));
#4088=CARTESIAN_POINT('Ctrl Pts',(-11.6251169246386,0.593998158860184,-5.89580760773948));
#4089=CARTESIAN_POINT('Ctrl Pts',(-11.6450883435803,0.619316987750228,-5.89325081894841));
#4090=CARTESIAN_POINT('Ctrl Pts',(-11.6644136094771,0.643816654094558,-5.89077675221468));
#4091=CARTESIAN_POINT('Ctrl Pts',(-11.6847525915489,0.667237341250066,-5.88827337457224));
#4092=CARTESIAN_POINT('Ctrl Pts',(-11.7059060210901,0.689460406258321,-5.88579242084807));
#4093=CARTESIAN_POINT('Ctrl Pts',(-11.7261027910912,0.710678437680429,-5.88342366775048));
#4094=CARTESIAN_POINT('Ctrl Pts',(-11.7476344282494,0.731426349304129,-5.88100685224014));
#4095=CARTESIAN_POINT('Ctrl Pts',(-11.7704316787271,0.751443261485303,-5.87859232221928));
#4096=CARTESIAN_POINT('Ctrl Pts',(-11.792944613224,0.771210532683476,-5.87620790501715));
#4097=CARTESIAN_POINT('Ctrl Pts',(-11.8166915647589,0.790264293271009,-5.87382571665301));
#4098=CARTESIAN_POINT('Ctrl Pts',(-11.8415590054149,0.808373164992864,-5.87149424468247));
#4099=CARTESIAN_POINT('Ctrl Pts',(-11.866288678916,0.826381712448536,-5.86917568921045));
#4100=CARTESIAN_POINT('Ctrl Pts',(-11.8921261252638,0.843455222096322,-5.86690728974473));
#4101=CARTESIAN_POINT('Ctrl Pts',(-11.9189171953938,0.859395040593982,-5.86473673242511));
#4102=CARTESIAN_POINT('Ctrl Pts',(-11.9455822675806,0.875259894398724,-5.86257638319934));
#4103=CARTESIAN_POINT('Ctrl Pts',(-11.9731915440691,0.890001198131698,-5.86051295798388));
#4104=CARTESIAN_POINT('Ctrl Pts',(-12.0015568587732,0.903459936989056,-5.85859347327646));
#4105=CARTESIAN_POINT('Ctrl Pts',(-12.0113696684317,0.90811590657827,-5.85792943911105));
#4106=CARTESIAN_POINT('Ctrl Pts',(-12.0212726736568,0.91261874057659,-5.85728263134725));
#4107=CARTESIAN_POINT('Ctrl Pts',(-12.0312572421975,0.916963043025268,-5.85665499654412));
#4108=CARTESIAN_POINT('Ctrl Pts',(-12.0588063180869,0.928949691958269,-5.85492324832167));
#4109=CARTESIAN_POINT('Ctrl Pts',(-12.0870049770799,0.93973768627278,-5.85335622415252));
#4110=CARTESIAN_POINT('Ctrl Pts',(-12.1156382920204,0.949227285060628,-5.85196428648677));
#4111=CARTESIAN_POINT('Ctrl Pts',(-12.1443073748145,0.958728737962493,-5.85057061005544));
#4112=CARTESIAN_POINT('Ctrl Pts',(-12.1734115519112,0.966928319492569,-5.84935245782604));
#4113=CARTESIAN_POINT('Ctrl Pts',(-12.2027184572862,0.973775525356251,-5.84832023113058));
#4114=CARTESIAN_POINT('Ctrl Pts',(-12.2320804477626,0.9806356011912,-5.84728606426737));
#4115=CARTESIAN_POINT('Ctrl Pts',(-12.2616452441127,0.986138143316237,-5.84643852252421));
#4116=CARTESIAN_POINT('Ctrl Pts',(-12.2911725495681,0.990284400605293,-5.84578806599426));
#4117=CARTESIAN_POINT('Ctrl Pts',(-12.3209050503466,0.994459471651339,-5.84513308921989));
#4118=CARTESIAN_POINT('Ctrl Pts',(-12.3505988485243,0.997259402232014,-5.84467794640146));
#4119=CARTESIAN_POINT('Ctrl Pts',(-12.3800123124227,0.998738326460704,-5.84443331722338));
#4120=CARTESIAN_POINT('Ctrl Pts',(-12.3968576798465,0.999585320276542,-5.84429321579222));
#4121=CARTESIAN_POINT('Ctrl Pts',(-12.4136112257704,1.,-5.84422216200635));
#4122=CARTESIAN_POINT('Ctrl Pts',(-12.4302293937643,1.,-5.84422216200635));
#4123=CARTESIAN_POINT('Origin',(-12.4302293937643,0.,0.));
#4124=CARTESIAN_POINT('',(-13.4302293937643,-3.9801020972289E-16,-4.5));
#4125=CARTESIAN_POINT('Origin',(-12.4302293937643,-2.75545529808154E-16,
-4.5));
#4126=CARTESIAN_POINT('',(-13.4302293937643,1.22464679914735E-16,-7.49879891330929E-33));
#4127=CARTESIAN_POINT('Origin',(-12.4302293937643,8.26636589424463E-16,
4.5));
#4128=CARTESIAN_POINT('Origin',(-12.4302293937643,4.5,-5.51091059616309E-16));
#4129=CARTESIAN_POINT('Origin',(-12.4302293937643,-2.75545529808154E-16,
-4.5));
#4130=CARTESIAN_POINT('Ctrl Pts',(-12.4302293937643,-6.08893299837349,-1.29488563599616));
#4131=CARTESIAN_POINT('Ctrl Pts',(-12.5942556094579,-6.08893299096372,-1.29488562495703));
#4132=CARTESIAN_POINT('Ctrl Pts',(-12.9435199759374,-6.10362004692185,-1.22941547699904));
#4133=CARTESIAN_POINT('Ctrl Pts',(-13.2353124874664,-6.14033341252253,-1.03140005307915));
#4134=CARTESIAN_POINT('Ctrl Pts',(-13.4654077531044,-6.17434194926064,-0.80247914861247));
#4135=CARTESIAN_POINT('Ctrl Pts',(-13.6642012577212,-6.21070412871452,-0.511738560164233));
#4136=CARTESIAN_POINT('Ctrl Pts',(-13.7305928319399,-6.2253945953946,-0.163672629624612));
#4137=CARTESIAN_POINT('Ctrl Pts',(-13.7305735234977,-6.22536971833509,0.163413942637349));
#4138=CARTESIAN_POINT('Ctrl Pts',(-13.6641961660918,-6.21065684408847,0.511524716651758));
#4139=CARTESIAN_POINT('Ctrl Pts',(-13.465346435092,-6.17428139683409,0.802173448767081));
#4140=CARTESIAN_POINT('Ctrl Pts',(-13.2353970954988,-6.14016146593015,1.0312922208101));
#4141=CARTESIAN_POINT('Ctrl Pts',(-13.0896053944545,-6.12196313951551,1.13039533120231));
#4142=CARTESIAN_POINT('Ctrl Pts',(-12.7690837661183,-6.09606085401061,1.2622143813522));
#4143=CARTESIAN_POINT('Ctrl Pts',(-12.5943834161953,-6.08887828006945,1.2946897058071));
#4144=CARTESIAN_POINT('Ctrl Pts',(-12.2661932789077,-6.08887357909258,1.29460046621699));
#4145=CARTESIAN_POINT('Ctrl Pts',(-12.0914931498336,-6.09604795264992,1.26198004011685));
#4146=CARTESIAN_POINT('Ctrl Pts',(-11.7709848415179,-6.12194030356741,1.12995676459186));
#4147=CARTESIAN_POINT('Ctrl Pts',(-11.6251708828575,-6.14012997800531,1.03077281364708));
#4148=CARTESIAN_POINT('Ctrl Pts',(-11.4025000109833,-6.17317174739286,0.808380882336614));
#4149=CARTESIAN_POINT('Ctrl Pts',(-11.2517604169044,-6.20030388726032,0.59559414446078));
#4150=CARTESIAN_POINT('Ctrl Pts',(-11.1346832359419,-6.22414177319952,0.217454422107557));
#4151=CARTESIAN_POINT('Ctrl Pts',(-11.1179113891857,-6.2277097295171,-0.121675282907419));
#4152=CARTESIAN_POINT('Ctrl Pts',(-11.1792551432517,-6.2148909110589,-0.376842015671391));
#4153=CARTESIAN_POINT('Ctrl Pts',(-11.2952430555643,-6.19246471770926,-0.656705157785398));
#4154=CARTESIAN_POINT('Ctrl Pts',(-11.3950443526158,-6.17434641001338,-0.801855766228741));
#4155=CARTESIAN_POINT('Ctrl Pts',(-11.6251511260733,-6.14020362776066,-1.03103200836982));
#4156=CARTESIAN_POINT('Ctrl Pts',(-11.7709033259227,-6.122014163478,-1.13030300160637));
#4157=CARTESIAN_POINT('Ctrl Pts',(-12.0914373624932,-6.09611196893258,-1.26225531127416));
#4158=CARTESIAN_POINT('Ctrl Pts',(-12.2662031836223,-6.08893299149969,-1.29488564095978));
#4159=CARTESIAN_POINT('Ctrl Pts',(-12.4302293937643,-6.08893299837349,-1.29488563599616));
#4160=CARTESIAN_POINT('Ctrl Pts',(-12.4302293937643,-6.00730670135932,-1.19652291995803));
#4161=CARTESIAN_POINT('Ctrl Pts',(-12.5835416075593,-6.00733185292099,-1.19656039090436));
#4162=CARTESIAN_POINT('Ctrl Pts',(-12.9099992478929,-6.02016943668172,-1.13400457500984));
#4163=CARTESIAN_POINT('Ctrl Pts',(-13.179481120053,-6.05208117737328,-0.947735263929781));
#4164=CARTESIAN_POINT('Ctrl Pts',(-13.3905508253865,-6.08150297834998,-0.734658226364409));
#4165=CARTESIAN_POINT('Ctrl Pts',(-13.5709920959587,-6.11274177608899,-0.466042577449154));
#4166=CARTESIAN_POINT('Ctrl Pts',(-13.6304639246011,-6.12529782064175,-0.149051739413726));
#4167=CARTESIAN_POINT('Ctrl Pts',(-13.6304533897943,-6.12527260806574,0.148787647638987));
#4168=CARTESIAN_POINT('Ctrl Pts',(-13.5709720447989,-6.11269507902186,0.465848644629128));
#4169=CARTESIAN_POINT('Ctrl Pts',(-13.3905041431794,-6.08144180450652,0.734326683901586));
#4170=CARTESIAN_POINT('Ctrl Pts',(-13.1795428364226,-6.05191130345156,0.947674493001592));
#4171=CARTESIAN_POINT('Ctrl Pts',(-13.0449586384788,-6.03611037539515,1.04079617562098));
#4172=CARTESIAN_POINT('Ctrl Pts',(-12.7469388659841,-6.01354168438538,1.16540284340237));
#4173=CARTESIAN_POINT('Ctrl Pts',(-12.5836962315238,-6.00726039156444,1.19631326107954));
#4174=CARTESIAN_POINT('Ctrl Pts',(-12.2768814243267,-6.00725251877471,1.19624527202557));
#4175=CARTESIAN_POINT('Ctrl Pts',(-12.1136335971426,-6.01353340392645,1.16513750020312));
#4176=CARTESIAN_POINT('Ctrl Pts',(-11.8156395078111,-6.03608069520521,1.04040354702773));
#4177=CARTESIAN_POINT('Ctrl Pts',(-11.6810080385117,-6.0518936089174,0.947061071249189));
#4178=CARTESIAN_POINT('Ctrl Pts',(-11.476775432527,-6.0804537040016,0.740195388112021));
#4179=CARTESIAN_POINT('Ctrl Pts',(-11.3397927474364,-6.1038110687889,0.543436243686021));
#4180=CARTESIAN_POINT('Ctrl Pts',(-11.2343328423298,-6.12419591144059,0.197848988748778));
#4181=CARTESIAN_POINT('Ctrl Pts',(-11.2192240525651,-6.12725896708914,-0.110526507186422));
#4182=CARTESIAN_POINT('Ctrl Pts',(-11.2744078114987,-6.11629204566253,-0.343438032428988));
#4183=CARTESIAN_POINT('Ctrl Pts',(-11.3792086385588,-6.09709227633881,-0.599872706676036));
#4184=CARTESIAN_POINT('Ctrl Pts',(-11.4699522513166,-6.08147950050026,-0.734057964386069));
#4185=CARTESIAN_POINT('Ctrl Pts',(-11.6809647607171,-6.05196881986237,-0.947385415737105));
#4186=CARTESIAN_POINT('Ctrl Pts',(-11.8155701530245,-6.03615792504545,-1.04071590511793));
#4187=CARTESIAN_POINT('Ctrl Pts',(-12.1135691209239,-6.01358992981694,-1.1654384548815));
#4188=CARTESIAN_POINT('Ctrl Pts',(-12.2768983357228,-6.00733003360885,-1.19650607159156));
#4189=CARTESIAN_POINT('Ctrl Pts',(-12.4302293937643,-6.00730670135932,-1.19652291995803));
#4190=CARTESIAN_POINT('Ctrl Pts',(-12.4302293937643,-5.92568040434515,-1.09816020391989));
#4191=CARTESIAN_POINT('Ctrl Pts',(-12.5728617871465,-5.92565520838872,-1.09812266683399));
#4192=CARTESIAN_POINT('Ctrl Pts',(-12.8764307452579,-5.93669281540111,-1.03868333620408));
#4193=CARTESIAN_POINT('Ctrl Pts',(-13.1237066796822,-5.96381552620845,-0.863916643031107));
#4194=CARTESIAN_POINT('Ctrl Pts',(-13.3156785658162,-5.98860458124536,-0.666696003113148));
#4195=CARTESIAN_POINT('Ctrl Pts',(-13.4779257102115,-6.01480861265757,-0.420423936232896));
#4196=CARTESIAN_POINT('Ctrl Pts',(-13.5302115977681,-6.0251142009875,-0.134359645298094));
#4197=CARTESIAN_POINT('Ctrl Pts',(-13.5301694517177,-6.02509693896035,0.134284106327718));
#4198=CARTESIAN_POINT('Ctrl Pts',(-13.4779135143473,-6.01477545935064,0.420354149772739));
#4199=CARTESIAN_POINT('Ctrl Pts',(-13.3155662884545,-5.98856196814462,0.666614474975836));
#4200=CARTESIAN_POINT('Ctrl Pts',(-13.1237490229197,-5.96369791624148,0.863960278040423));
#4201=CARTESIAN_POINT('Ctrl Pts',(-13.0002570596326,-5.95026526779515,0.951291302906749));
#4202=CARTESIAN_POINT('Ctrl Pts',(-12.7248192878539,-5.93103075476377,1.06853916455731));
#4203=CARTESIAN_POINT('Ctrl Pts',(-12.5729580288434,-5.92565006141073,1.09800243214524));
#4204=CARTESIAN_POINT('Ctrl Pts',(-12.287577286871,-5.92565044560247,1.09790991870327));
#4205=CARTESIAN_POINT('Ctrl Pts',(-12.1357205964749,-5.9310187003764,1.06838177460848));
#4206=CARTESIAN_POINT('Ctrl Pts',(-11.8602821295538,-5.9502584447237,0.950895885550572));
#4207=CARTESIAN_POINT('Ctrl Pts',(-11.736788079086,-5.96366715170961,0.863629609851932));
#4208=CARTESIAN_POINT('Ctrl Pts',(-11.5510151221346,-5.98777821987636,0.67188359125213));
#4209=CARTESIAN_POINT('Ctrl Pts',(-11.427751170242,-6.00731764764785,0.491487465397297));
#4210=CARTESIAN_POINT('Ctrl Pts',(-11.3339016795611,-6.02427343221154,0.178379449022163));
#4211=CARTESIAN_POINT('Ctrl Pts',(-11.3206116198576,-6.02677974461079,-0.0997509032157466));
#4212=CARTESIAN_POINT('Ctrl Pts',(-11.3695095553554,-6.01770990863714,-0.310016341778994));
#4213=CARTESIAN_POINT('Ctrl Pts',(-11.463356556165,-6.00165061145685,-0.543287387943066));
#4214=CARTESIAN_POINT('Ctrl Pts',(-11.5448540553375,-5.98861113270541,-0.666319219911386));
#4215=CARTESIAN_POINT('Ctrl Pts',(-11.7368736448428,-5.96369271832399,-0.86381896190319));
#4216=CARTESIAN_POINT('Ctrl Pts',(-11.8602625947015,-5.95028583599656,-0.951226144039803));
#4217=CARTESIAN_POINT('Ctrl Pts',(-12.1357218721558,-5.93105211422019,-1.06859726081973));
#4218=CARTESIAN_POINT('Ctrl Pts',(-12.2876158778903,-5.92565703091211,-1.09817708202523));
#4219=CARTESIAN_POINT('Ctrl Pts',(-12.4302293937643,-5.92568040434515,-1.09816020391989));
#4220=CARTESIAN_POINT('Ctrl Pts',(-12.4302293937643,-5.84405410733098,-0.999797487881759));
#4221=CARTESIAN_POINT('Ctrl Pts',(-12.5621477450218,-5.84405415920521,-0.999797565164297));
#4222=CARTESIAN_POINT('Ctrl Pts',(-12.8429100734364,-5.85324223577186,-0.943272328695468));
#4223=CARTESIAN_POINT('Ctrl Pts',(-13.0678752452747,-5.87556330684772,-0.780252034917407));
#4224=CARTESIAN_POINT('Ctrl Pts',(-13.2408216561416,-5.89576568026994,-0.598875247154049));
#4225=CARTESIAN_POINT('Ctrl Pts',(-13.3847163804241,-5.91684622568096,-0.374727862499088));
#4226=CARTESIAN_POINT('Ctrl Pts',(-13.4300828356746,-5.9250175284374,-0.119738838882957));
#4227=CARTESIAN_POINT('Ctrl Pts',(-13.4300495107861,-5.92499992114235,0.119657666867655));
#4228=CARTESIAN_POINT('Ctrl Pts',(-13.3846891981801,-5.91681364468555,0.374677864062464));
#4229=CARTESIAN_POINT('Ctrl Pts',(-13.2407241090043,-5.89572242317792,0.598767551759252));
#4230=CARTESIAN_POINT('Ctrl Pts',(-13.0678946927086,-5.87544771048421,0.780342663782052));
#4231=CARTESIAN_POINT('Ctrl Pts',(-12.9556103681747,-5.86441249466429,0.861692036369364));
#4232=CARTESIAN_POINT('Ctrl Pts',(-12.7026743579198,-5.84851157544137,0.97172768796908));
#4233=CARTESIAN_POINT('Ctrl Pts',(-12.562270904212,-5.84403216401073,0.999625910198263));
#4234=CARTESIAN_POINT('Ctrl Pts',(-12.2982654232083,-5.84402936293972,0.999554701162274));
#4235=CARTESIAN_POINT('Ctrl Pts',(-12.1578611066837,-5.84850415183514,0.971539132528016));
#4236=CARTESIAN_POINT('Ctrl Pts',(-11.9049368100215,-5.86439879239718,0.861342614374135));
#4237=CARTESIAN_POINT('Ctrl Pts',(-11.7926253019556,-5.87543077095699,0.779917537607569));
#4238=CARTESIAN_POINT('Ctrl Pts',(-11.625290585729,-5.89506012639956,0.603698245665789));
#4239=CARTESIAN_POINT('Ctrl Pts',(-11.5157835877516,-5.91082482988569,0.439329318518403));
#4240=CARTESIAN_POINT('Ctrl Pts',(-11.4335513810015,-5.92432754293507,0.158773855738042));
#4241=CARTESIAN_POINT('Ctrl Pts',(-11.421924195087,-5.92632901567582,-0.0886016883305396));
#4242=CARTESIAN_POINT('Ctrl Pts',(-11.4646622835325,-5.91911102355411,-0.276612379375412));
#4243=CARTESIAN_POINT('Ctrl Pts',(-11.5473219245805,-5.90627825155154,-0.486454645997929));
#4244=CARTESIAN_POINT('Ctrl Pts',(-11.6197619612107,-5.89574422490846,-0.59852134856752));
#4245=CARTESIAN_POINT('Ctrl Pts',(-11.792687167393,-5.87545795902179,-0.78017227495977));
#4246=CARTESIAN_POINT('Ctrl Pts',(-11.904929391659,-5.86442961621768,-0.861638933002959));
#4247=CARTESIAN_POINT('Ctrl Pts',(-12.1578536058814,-5.84853009367097,-0.971780433068657));
#4248=CARTESIAN_POINT('Ctrl Pts',(-12.2983110036412,-5.84405415545294,-0.999797453132582));
#4249=CARTESIAN_POINT('Ctrl Pts',(-12.4302293937643,-5.84405410733098,-0.999797487881759));
#4250=CARTESIAN_POINT('',(-12.4302293937643,-5.84422216200635,-1.));
#4251=CARTESIAN_POINT('',(-12.4302293937643,-6.08890895085005,-1.29485665783831));
#4252=CARTESIAN_POINT('',(-13.4302293937643,-5.9251719038059,1.0785270517389E-16));
#4253=CARTESIAN_POINT('Ctrl Pts',(-12.4302293937643,-5.84422216200635,-1.));
#4254=CARTESIAN_POINT('Ctrl Pts',(-12.4944982458915,-5.84422216200635,-1.));
#4255=CARTESIAN_POINT('Ctrl Pts',(-12.5587518483679,-5.84562231156004,-0.993793077287905));
#4256=CARTESIAN_POINT('Ctrl Pts',(-12.6840917070905,-5.84953577508847,-0.969312352511264));
#4257=CARTESIAN_POINT('Ctrl Pts',(-12.7449916575148,-5.85204625647294,-0.951276694198755));
#4258=CARTESIAN_POINT('Ctrl Pts',(-12.864337458649,-5.85877465283481,-0.903230714929781));
#4259=CARTESIAN_POINT('Ctrl Pts',(-12.9223384459871,-5.8632652060475,-0.872966477219125));
#4260=CARTESIAN_POINT('Ctrl Pts',(-13.0310521006909,-5.87276344316928,-0.801996314727874));
#4261=CARTESIAN_POINT('Ctrl Pts',(-13.0816795448316,-5.87769727434892,-0.761443393429155));
#4262=CARTESIAN_POINT('Ctrl Pts',(-13.1735637062492,-5.88774709930129,-0.671936344908102));
#4263=CARTESIAN_POINT('Ctrl Pts',(-13.2147234026552,-5.89313164041396,-0.623382463895755));
#4264=CARTESIAN_POINT('Ctrl Pts',(-13.2878087312711,-5.90320437241943,-0.518368774693091));
#4265=CARTESIAN_POINT('Ctrl Pts',(-13.3194196283319,-5.90778220806811,-0.462062726244169));
#4266=CARTESIAN_POINT('Ctrl Pts',(-13.3714221289722,-5.91556605482255,-0.343975848624026));
#4267=CARTESIAN_POINT('Ctrl Pts',(-13.3917043040785,-5.91892406306771,-0.282400092474657));
#4268=CARTESIAN_POINT('Ctrl Pts',(-13.420000040749,-5.92359300815781,-0.156508651779502));
#4269=CARTESIAN_POINT('Ctrl Pts',(-13.4280159105558,-5.92484933356782,-0.0925661452570473));
#4270=CARTESIAN_POINT('Ctrl Pts',(-13.4300968211925,-5.92515214681615,-0.0188017619570889));
#4271=CARTESIAN_POINT('Ctrl Pts',(-13.4302293937643,-5.9251709568609,-0.00940098878205599));
#4272=CARTESIAN_POINT('Ctrl Pts',(-13.4302293937643,-5.9251719038059,-4.20390922051782E-16));
#4273=CARTESIAN_POINT('Ctrl Pts',(-13.4302293937643,-5.9251719038059,-4.20390922051782E-16));
#4274=CARTESIAN_POINT('Ctrl Pts',(-13.4302293937643,-5.92517721135784,0.0526917995608284));
#4275=CARTESIAN_POINT('Ctrl Pts',(-13.4260601515651,-5.92458148056859,0.105390376886493));
#4276=CARTESIAN_POINT('Ctrl Pts',(-13.4077283650324,-5.92160517649706,0.220319257946971));
#4277=CARTESIAN_POINT('Ctrl Pts',(-13.3917600419347,-5.91889366817302,0.281942156475162));
#4278=CARTESIAN_POINT('Ctrl Pts',(-13.3480477817509,-5.91202032426913,0.402198254109568));
#4279=CARTESIAN_POINT('Ctrl Pts',(-13.3202407961492,-5.90795462801506,0.460471360524695));
#4280=CARTESIAN_POINT('Ctrl Pts',(-13.2535116311086,-5.89846585980263,0.57133537793989));
#4281=CARTESIAN_POINT('Ctrl Pts',(-13.2146990232233,-5.89303091664152,0.623545922817736));
#4282=CARTESIAN_POINT('Ctrl Pts',(-13.1291961220027,-5.8825630261041,0.717879440332942));
#4283=CARTESIAN_POINT('Ctrl Pts',(-13.0830058863189,-5.87774668100827,0.76012306424411));
#4284=CARTESIAN_POINT('Ctrl Pts',(-12.9826770102536,-5.86824548138472,0.83594569086839));
#4285=CARTESIAN_POINT('Ctrl Pts',(-12.9286733506225,-5.86357871145779,0.869229122032554));
#4286=CARTESIAN_POINT('Ctrl Pts',(-12.814646447115,-5.85546947246655,0.925361834437775));
#4287=CARTESIAN_POINT('Ctrl Pts',(-12.7550536475759,-5.85234789442664,0.947920256643328));
#4288=CARTESIAN_POINT('Ctrl Pts',(-12.6077286786872,-5.84664782631375,0.988134290189823));
#4289=CARTESIAN_POINT('Ctrl Pts',(-12.5190391995663,-5.84434890472074,0.999996557140233));
#4290=CARTESIAN_POINT('Ctrl Pts',(-12.3414508870207,-5.84439252370977,1.00000344312345));
#4291=CARTESIAN_POINT('Ctrl Pts',(-12.2527245841438,-5.84675093906306,0.988135859292573));
#4292=CARTESIAN_POINT('Ctrl Pts',(-12.1053731550729,-5.85253966996574,0.947909320920726));
#4293=CARTESIAN_POINT('Ctrl Pts',(-12.0457787622019,-5.85569317128686,0.925347745846651));
#4294=CARTESIAN_POINT('Ctrl Pts',(-11.9317032574863,-5.86385480068626,0.869186241970665));
#4295=CARTESIAN_POINT('Ctrl Pts',(-11.8776535063375,-5.86854502214797,0.835865276146026));
#4296=CARTESIAN_POINT('Ctrl Pts',(-11.7771843657185,-5.87810913986364,0.759903727134754));
#4297=CARTESIAN_POINT('Ctrl Pts',(-11.7309014155548,-5.88301655964537,0.717535821849503));
#4298=CARTESIAN_POINT('Ctrl Pts',(-11.6446884611433,-5.89355171795038,0.622305619278858));
#4299=CARTESIAN_POINT('Ctrl Pts',(-11.6053836802498,-5.89886076131314,0.56919270515609));
#4300=CARTESIAN_POINT('Ctrl Pts',(-11.5549487679018,-5.90590573411597,0.484702051427652));
#4301=CARTESIAN_POINT('Ctrl Pts',(-11.5396848313392,-5.90809410537879,0.456052361783949));
#4302=CARTESIAN_POINT('Ctrl Pts',(-11.4984673381252,-5.91423227905847,0.368691539381281));
#4303=CARTESIAN_POINT('Ctrl Pts',(-11.4766739314384,-5.91795523502758,0.308013717888738));
#4304=CARTESIAN_POINT('Ctrl Pts',(-11.445711632252,-5.92296069604394,0.185827526072649));
#4305=CARTESIAN_POINT('Ctrl Pts',(-11.436138601018,-5.9242390513156,0.124800058789788));
#4306=CARTESIAN_POINT('Ctrl Pts',(-11.428157368614,-5.92535267058096,-0.000936975829386351));
#4307=CARTESIAN_POINT('Ctrl Pts',(-11.4302996049242,-5.92520408286643,-0.0656208398590233));
#4308=CARTESIAN_POINT('Ctrl Pts',(-11.447092733453,-5.92251839001045,-0.19408607762655));
#4309=CARTESIAN_POINT('Ctrl Pts',(-11.4617712884571,-5.91996522088789,-0.25749448426409));
#4310=CARTESIAN_POINT('Ctrl Pts',(-11.5032325236537,-5.91324612004577,-0.380667291322442));
#4311=CARTESIAN_POINT('Ctrl Pts',(-11.5299666236449,-5.90927771739317,-0.44018443126589));
#4312=CARTESIAN_POINT('Ctrl Pts',(-11.5783475393985,-5.90247649310005,-0.524730963460824));
#4313=CARTESIAN_POINT('Ctrl Pts',(-11.595748617846,-5.90006780571956,-0.551983456838474));
#4314=CARTESIAN_POINT('Ctrl Pts',(-11.651223457358,-5.89258038162579,-0.630234975445558));
#4315=CARTESIAN_POINT('Ctrl Pts',(-11.6928573009781,-5.88719076659233,-0.678478398391647));
#4316=CARTESIAN_POINT('Ctrl Pts',(-11.785608298049,-5.87706819763353,-0.767238038743982));
#4317=CARTESIAN_POINT('Ctrl Pts',(-11.8366404907297,-5.87210453132499,-0.807369546161976));
#4318=CARTESIAN_POINT('Ctrl Pts',(-11.946000874798,-5.86260028948649,-0.877358832991084));
#4319=CARTESIAN_POINT('Ctrl Pts',(-12.0042344687816,-5.85810609494132,-0.907081501893602));
#4320=CARTESIAN_POINT('Ctrl Pts',(-12.1237240476056,-5.8514570651785,-0.953952809540106));
#4321=CARTESIAN_POINT('Ctrl Pts',(-12.1845405832366,-5.849045354789,-0.971400470233401));
#4322=CARTESIAN_POINT('Ctrl Pts',(-12.307144058756,-5.84544554810484,-0.994307498142081));
#4323=CARTESIAN_POINT('Ctrl Pts',(-12.3686784358337,-5.84422216200635,-1.));
#4324=CARTESIAN_POINT('Ctrl Pts',(-12.4302293937643,-5.84422216200635,-1.));
#4325=CARTESIAN_POINT('Origin',(-12.4302293937643,0.,0.));
#4326=CARTESIAN_POINT('',(-13.4302293937643,-4.5,1.22464679914735E-16));
#4327=CARTESIAN_POINT('Origin',(-12.4302293937643,-4.5,0.));
#4328=CARTESIAN_POINT('',(-13.4302293937643,0.,-1.22464679914735E-16));
#4329=CARTESIAN_POINT('Origin',(-12.4302293937643,-4.5,0.));
#4330=CARTESIAN_POINT('Origin',(-14.3242463976144,0.,-5.96248981933611));
#4331=CARTESIAN_POINT('',(-14.3242463976144,-7.30194407219864E-16,5.96248981933611));
#4332=CARTESIAN_POINT('Origin',(-14.3242463976144,0.,0.));
#4333=CARTESIAN_POINT('',(-14.3242463976144,-4.4393205576042E-16,3.62498032958974));
#4334=CARTESIAN_POINT('Origin',(-14.3242463976144,0.,0.));
#4335=CARTESIAN_POINT('Origin',(-14.2019363570046,0.,0.));
#4336=CARTESIAN_POINT('',(-14.2019363570046,-7.46272655961369E-16,6.09377868362497));
#4337=CARTESIAN_POINT('Origin',(-10.6585224305239,0.,0.));
#4338=CARTESIAN_POINT('',(-10.5362123899142,-7.30194407219864E-16,5.96248981933611));
#4339=CARTESIAN_POINT('',(-10.6585224305239,7.46272655961369E-16,6.09377868362497));
#4340=CARTESIAN_POINT('Origin',(-10.5362123899142,0.,0.));
#4341=CARTESIAN_POINT('Origin',(-10.5362123899142,0.,-3.62498032958974));
#4342=CARTESIAN_POINT('',(-10.5362123899142,-4.4393205576042E-16,3.62498032958974));
#4343=CARTESIAN_POINT('Origin',(-10.5362123899142,0.,0.));
#4344=CARTESIAN_POINT('Origin',(-10.6678019790643,0.,0.));
#4345=CARTESIAN_POINT('',(-10.7993915682143,-3.88369225985197E-16,3.17127539348974));
#4346=CARTESIAN_POINT('Origin',(-10.7993915682143,0.,0.));
#4347=CARTESIAN_POINT('',(-10.6678019790643,-4.16150640872808E-16,3.39812786153974));
#4348=CARTESIAN_POINT('Origin',(-12.4302293937643,0.,0.));
#4349=CARTESIAN_POINT('',(-14.0610672193142,-3.88369225985197E-16,3.17127539348974));
#4350=CARTESIAN_POINT('Origin',(-14.0610672193142,0.,0.));
#4351=CARTESIAN_POINT('',(-12.4302293937643,-3.88369225985197E-16,3.17127539348974));
#4352=CARTESIAN_POINT('Origin',(-14.1926568084643,0.,0.));
#4353=CARTESIAN_POINT('',(-14.1926568084643,4.16150640872808E-16,3.39812786153974));
#4600=UNCERTAINTY_MEASURE_WITH_UNIT(LENGTH_MEASURE(0.01),#4614,
'DISTANCE_ACCURACY_VALUE',
'Maximum model space distance between geometric entities at asserted c
onnectivities');
#4603=UNCERTAINTY_MEASURE_WITH_UNIT(LENGTH_MEASURE(0.01),#4614,
'DISTANCE_ACCURACY_VALUE',
'Maximum model space distance between geometric entities at asserted c
onnectivities');
#4610=(
GEOMETRIC_REPRESENTATION_CONTEXT(3)
GLOBAL_UNCERTAINTY_ASSIGNED_CONTEXT((#4600))
GLOBAL_UNIT_ASSIGNED_CONTEXT((#4614,#4616,#4617))
REPRESENTATION_CONTEXT('','3D')
);
#4613=(
GEOMETRIC_REPRESENTATION_CONTEXT(3)
GLOBAL_UNCERTAINTY_ASSIGNED_CONTEXT((#4603))
GLOBAL_UNIT_ASSIGNED_CONTEXT((#4614,#4616,#4617))
REPRESENTATION_CONTEXT('','3D')
);
#4614=(
LENGTH_UNIT()
NAMED_UNIT(*)
SI_UNIT(.MILLI.,.METRE.)
);
#4616=(
NAMED_UNIT(*)
PLANE_ANGLE_UNIT()
SI_UNIT($,.RADIAN.)
);
#4617=(
NAMED_UNIT(*)
SI_UNIT($,.STERADIAN.)
SOLID_ANGLE_UNIT()
);
#4624=SHAPE_DEFINITION_REPRESENTATION(#4633,#4650);
#4633=PRODUCT_DEFINITION_SHAPE('',$,#4660);
#4650=SHAPE_REPRESENTATION('',(#1812),#4610);
#4653=PRODUCT_DEFINITION_CONTEXT('part definition',#4682,'design');
#4660=PRODUCT_DEFINITION('Locker','Locker',#4669,#4653);
#4669=PRODUCT_DEFINITION_FORMATION('',$,#4690);
#4682=APPLICATION_CONTEXT(
'Core Data for Automotive Mechanical Design Process');
#4683=PRODUCT_CONTEXT('part definition',#4682,'mechanical');
#4690=PRODUCT('Locker','Locker',$,(#4683));
#4695=PRESENTATION_STYLE_ASSIGNMENT((#4700));
#4700=SURFACE_STYLE_USAGE(.BOTH.,#4705);
#4705=SURFACE_SIDE_STYLE('',(#4710));
#4710=SURFACE_STYLE_FILL_AREA(#4715);
#4715=FILL_AREA_STYLE('Opaque(255,255,255)',(#4720));
#4720=FILL_AREA_STYLE_COLOUR('Opaque(255,255,255)',#4725);
#4725=COLOUR_RGB('Opaque(255,255,255)', 0.66274510, 0.83137255, 0.94901961);
ENDSEC;
END-ISO-10303-21;
